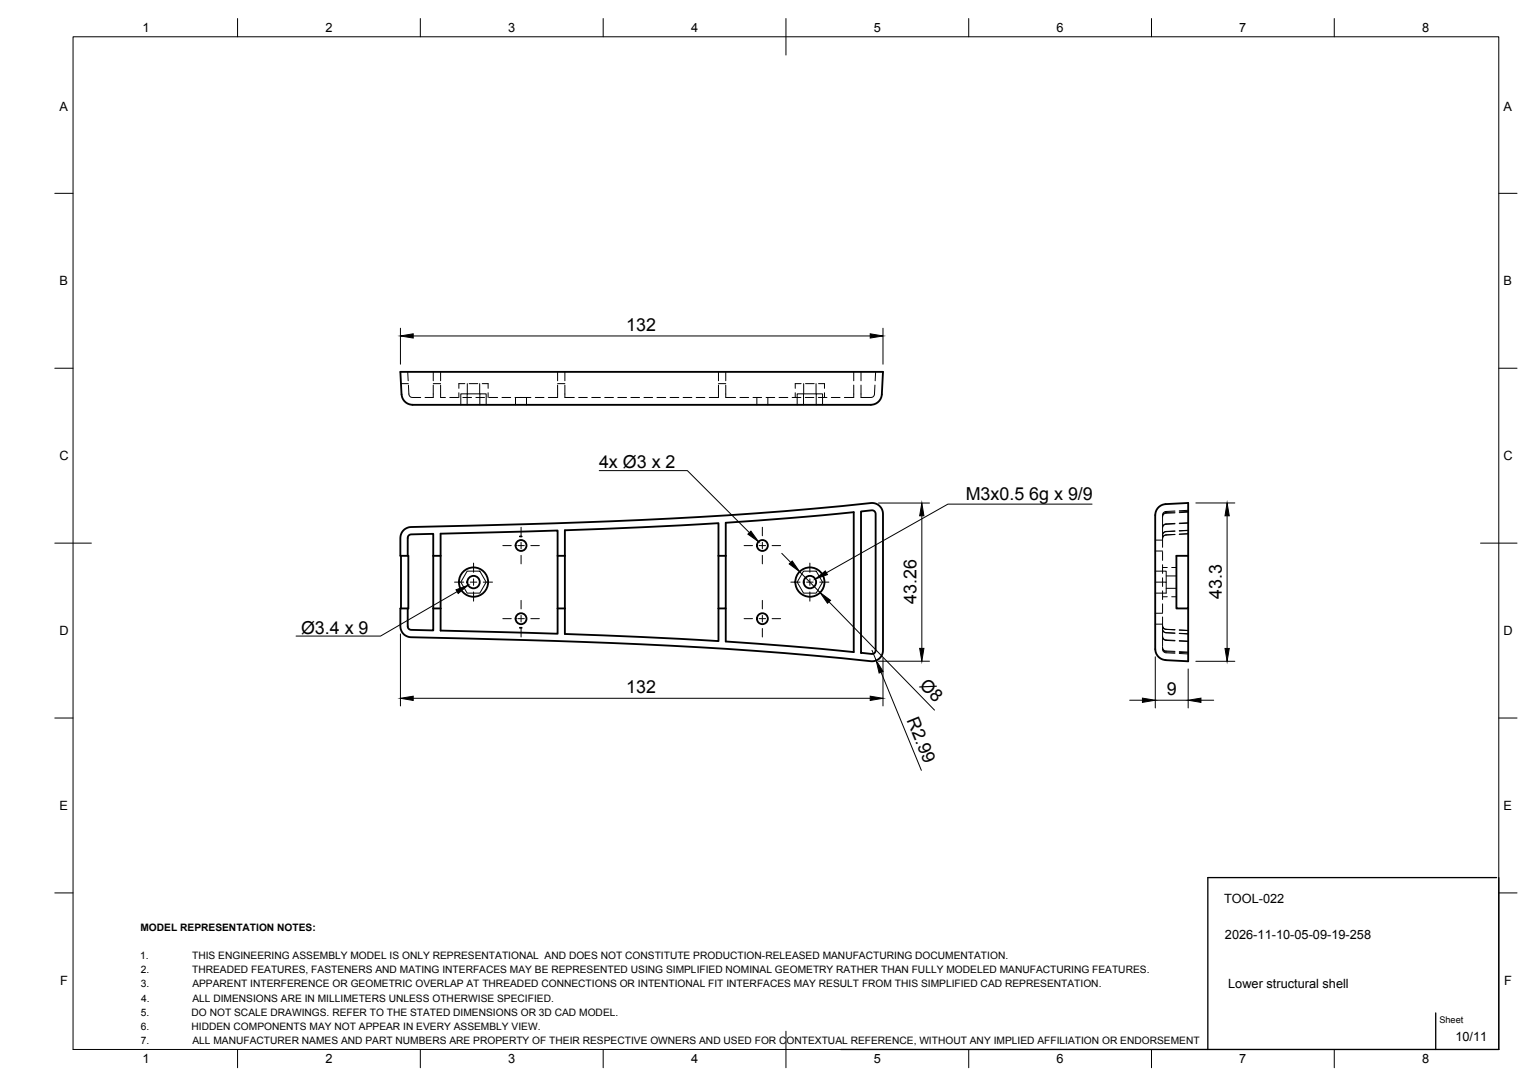
ISO-10303-21;
HEADER;
/* Generated by software containing ST-Developer
 * from STEP Tools, Inc. (www.steptools.com) 
 */

FILE_DESCRIPTION(
/* description */ (''),
/* implementation_level */ '2;1');

FILE_NAME(
/* name */ 'Lower structural shell.step',
/* time_stamp */ '2026-11-10T08:27:36-08:00',
/* author */ (''),
/* organization */ (''),
/* preprocessor_version */ 'ST-DEVELOPER v20.2',
/* originating_system */ 'Autodesk Translation Framework v15.17.0.0',
/* authorisation */ '');

FILE_SCHEMA (('AUTOMOTIVE_DESIGN { 1 0 10303 214 3 1 1 }'));
ENDSEC;

DATA;
#10=MECHANICAL_DESIGN_GEOMETRIC_PRESENTATION_REPRESENTATION('',(#571),#19090);
#84=SPHERICAL_SURFACE('',#7214,0.0999999999999999);
#85=SPHERICAL_SURFACE('',#7217,0.0999999999999997);
#86=SPHERICAL_SURFACE('',#7221,0.0999999999999998);
#87=SPHERICAL_SURFACE('',#7225,0.1);
#88=SPHERICAL_SURFACE('',#7230,0.3);
#89=SPHERICAL_SURFACE('',#7234,0.3);
#90=SPHERICAL_SURFACE('',#7238,0.3);
#91=SPHERICAL_SURFACE('',#7243,0.3);
#124=B_SPLINE_SURFACE_WITH_KNOTS('',3,3,((#12291,#12292,#12293,#12294),
(#12295,#12296,#12297,#12298),(#12299,#12300,#12301,#12302),(#12303,#12304,
#12305,#12306)),.UNSPECIFIED.,.F.,.F.,.F.,(4,4),(4,4),(0.0600191787356395,
0.326709122771036),(0.0105314009467253,0.683686938235975),.UNSPECIFIED.);
#125=B_SPLINE_SURFACE_WITH_KNOTS('',3,3,((#12311,#12312,#12313,#12314),
(#12315,#12316,#12317,#12318),(#12319,#12320,#12321,#12322),(#12323,#12324,
#12325,#12326)),.UNSPECIFIED.,.F.,.F.,.F.,(4,4),(4,4),(0.0251675824878611,
0.0470055662028096),(0.0103663370325175,0.682341693918943),
 .UNSPECIFIED.);
#126=B_SPLINE_SURFACE_WITH_KNOTS('',3,3,((#12336,#12337,#12338,#12339),
(#12340,#12341,#12342,#12343),(#12344,#12345,#12346,#12347),(#12348,#12349,
#12350,#12351),(#12352,#12353,#12354,#12355)),.UNSPECIFIED.,.F.,.F.,.F.,
(4,1,4),(4,4),(0.,0.571428571428571,1.),(0.796205213256333,4.31873271634551),
 .UNSPECIFIED.);
#127=B_SPLINE_SURFACE_WITH_KNOTS('',3,3,((#12360,#12361,#12362,#12363),
(#12364,#12365,#12366,#12367),(#12368,#12369,#12370,#12371),(#12372,#12373,
#12374,#12375),(#12376,#12377,#12378,#12379)),.UNSPECIFIED.,.F.,.F.,.F.,
(4,1,4),(4,4),(0.,0.571428571428571,1.),(0.335767855111383,0.605460332260614),
 .UNSPECIFIED.);
#128=B_SPLINE_SURFACE_WITH_KNOTS('',3,3,((#12398,#12399,#12400,#12401),
(#12402,#12403,#12404,#12405),(#12406,#12407,#12408,#12409),(#12410,#12411,
#12412,#12413),(#12414,#12415,#12416,#12417)),.UNSPECIFIED.,.F.,.F.,.F.,
(4,1,4),(4,4),(0.,0.571428571428571,1.),(8.8675541747208,12.3900816778099),
 .UNSPECIFIED.);
#129=B_SPLINE_SURFACE_WITH_KNOTS('',3,3,((#12422,#12423,#12424,#12425),
(#12426,#12427,#12428,#12429),(#12430,#12431,#12432,#12433),(#12434,#12435,
#12436,#12437)),.UNSPECIFIED.,.F.,.F.,.F.,(4,4),(4,4),(0.673290877228964,
0.939980821264432),(0.010531400969624,0.683686938235975),.UNSPECIFIED.);
#130=B_SPLINE_SURFACE_WITH_KNOTS('',3,3,((#12438,#12439,#12440,#12441),
(#12442,#12443,#12444,#12445),(#12446,#12447,#12448,#12449),(#12450,#12451,
#12452,#12453)),.UNSPECIFIED.,.F.,.F.,.F.,(4,4),(4,4),(0.952994433797115,
0.974832417512139),(0.0103663370325174,0.682341693895801),.UNSPECIFIED.);
#131=B_SPLINE_SURFACE_WITH_KNOTS('',3,3,((#12537,#12538,#12539,#12540),
(#12541,#12542,#12543,#12544),(#12545,#12546,#12547,#12548),(#12549,#12550,
#12551,#12552)),.UNSPECIFIED.,.F.,.F.,.F.,(4,4),(4,4),(0.341076481775573,
0.660379921919131),(0.0113804342297301,0.684288445414502),.UNSPECIFIED.);
#132=B_SPLINE_SURFACE_WITH_KNOTS('',3,3,((#12557,#12558,#12559,#12560),
(#12561,#12562,#12563,#12564),(#12565,#12566,#12567,#12568),(#12569,#12570,
#12571,#12572),(#12573,#12574,#12575,#12576)),.UNSPECIFIED.,.F.,.F.,.F.,
(4,1,4),(4,4),(0.,0.571428571428571,1.),(4.5128966022766,8.72381854299666),
 .UNSPECIFIED.);
#133=B_SPLINE_SURFACE_WITH_KNOTS('',3,3,((#12586,#12587,#12588,#12589),
(#12590,#12591,#12592,#12593),(#12594,#12595,#12596,#12597),(#12598,#12599,
#12600,#12601),(#12602,#12603,#12604,#12605)),.UNSPECIFIED.,.F.,.F.,.F.,
(4,1,4),(4,4),(0.,0.571428571428571,1.),(4.46246834806959,8.67339028878965),
 .UNSPECIFIED.);
#134=B_SPLINE_SURFACE_WITH_KNOTS('',3,3,((#12610,#12611,#12612,#12613),
(#12614,#12615,#12616,#12617),(#12618,#12619,#12620,#12621),(#12622,#12623,
#12624,#12625)),.UNSPECIFIED.,.F.,.F.,.F.,(4,4),(4,4),(0.33962007808087,
0.658923518224427),(0.0113804342297301,0.68428844541339),.UNSPECIFIED.);
#135=B_SPLINE_SURFACE_WITH_KNOTS('',3,3,((#12697,#12698,#12699,#12700),
(#12701,#12702,#12703,#12704),(#12705,#12706,#12707,#12708),(#12709,#12710,
#12711,#12712)),.UNSPECIFIED.,.F.,.F.,.F.,(4,4),(4,4),(0.67474627241906,
0.91907102854965),(0.0117551961069005,0.684448842095107),.UNSPECIFIED.);
#136=B_SPLINE_SURFACE_WITH_KNOTS('',3,3,((#12717,#12718,#12719,#12720),
(#12721,#12722,#12723,#12724),(#12725,#12726,#12727,#12728),(#12729,#12730,
#12731,#12732),(#12733,#12734,#12735,#12736)),.UNSPECIFIED.,.F.,.F.,.F.,
(4,1,4),(4,4),(0.,0.571428571428571,1.),(8.92068531110742,12.1251256661408),
 .UNSPECIFIED.);
#137=B_SPLINE_SURFACE_WITH_KNOTS('',3,3,((#12737,#12738,#12739,#12740),
(#12741,#12742,#12743,#12744),(#12745,#12746,#12747,#12748),(#12749,#12750,
#12751,#12752),(#12753,#12754,#12755,#12756)),.UNSPECIFIED.,.F.,.F.,.F.,
(4,1,4),(4,4),(0.,0.571428571428571,1.),(1.06116122492545,4.26560157995882),
 .UNSPECIFIED.);
#138=B_SPLINE_SURFACE_WITH_KNOTS('',3,3,((#12761,#12762,#12763,#12764),
(#12765,#12766,#12767,#12768),(#12769,#12770,#12771,#12772),(#12773,#12774,
#12775,#12776)),.UNSPECIFIED.,.F.,.F.,.F.,(4,4),(4,4),(0.0809289714503497,
0.325253727580939),(0.011755196108102,0.684448842095106),.UNSPECIFIED.);
#139=B_SPLINE_SURFACE_WITH_KNOTS('',3,3,((#12851,#12852,#12853,#12854),
(#12855,#12856,#12857,#12858),(#12859,#12860,#12861,#12862),(#12863,#12864,
#12865,#12866)),.UNSPECIFIED.,.F.,.F.,.F.,(4,4),(4,4),(0.932204931312898,
0.977820042778932),(0.0118590921259657,0.68448768567755),.UNSPECIFIED.);
#140=B_SPLINE_SURFACE_WITH_KNOTS('',3,3,((#12876,#12877,#12878,#12879),
(#12880,#12881,#12882,#12883),(#12884,#12885,#12886,#12887),(#12888,#12889,
#12890,#12891),(#12892,#12893,#12894,#12895)),.UNSPECIFIED.,.F.,.F.,.F.,
(4,1,4),(4,4),(0.,0.571428571428571,1.),(12.3228618033436,12.893479658151),
 .UNSPECIFIED.);
#141=B_SPLINE_SURFACE_WITH_KNOTS('',3,3,((#12909,#12910,#12911,#12912),
(#12913,#12914,#12915,#12916),(#12917,#12918,#12919,#12920),(#12921,#12922,
#12923,#12924)),.UNSPECIFIED.,.F.,.F.,.F.,(4,4),(4,4),(0.0221799572210682,
0.0677950686870383),(0.0118590921467069,0.68448768567755),.UNSPECIFIED.);
#142=B_SPLINE_SURFACE_WITH_KNOTS('',3,3,((#12934,#12935,#12936,#12937),
(#12938,#12939,#12940,#12941),(#12942,#12943,#12944,#12945),(#12946,#12947,
#12948,#12949),(#12950,#12951,#12952,#12953)),.UNSPECIFIED.,.F.,.F.,.F.,
(4,1,4),(4,4),(0.,0.571428571428571,1.),(0.29280723291527,0.863425087722636),
 .UNSPECIFIED.);
#143=B_SPLINE_SURFACE_WITH_KNOTS('',3,3,((#12967,#12968,#12969,#12970),
(#12971,#12972,#12973,#12974),(#12975,#12976,#12977,#12978),(#12979,#12980,
#12981,#12982),(#12983,#12984,#12985,#12986)),.UNSPECIFIED.,.F.,.F.,.F.,
(4,1,4),(4,4),(0.,0.571428571428571,1.),(0.00866835330220971,0.617725317592517),
 .UNSPECIFIED.);
#144=B_SPLINE_SURFACE_WITH_KNOTS('',3,3,((#12993,#12994,#12995,#12996),
(#12997,#12998,#12999,#13000),(#13001,#13002,#13003,#13004),(#13005,#13006,
#13007,#13008),(#13009,#13010,#13011,#13012),(#13013,#13014,#13015,#13016)),
 .UNSPECIFIED.,.F.,.F.,.F.,(4,1,1,4),(4,4),(0.,0.285714285714286,0.571428571428571,
1.),(0.00654045782928703,0.615688454110788),.UNSPECIFIED.);
#145=B_SPLINE_SURFACE_WITH_KNOTS('',3,3,((#13021,#13022,#13023,#13024),
(#13025,#13026,#13027,#13028),(#13029,#13030,#13031,#13032),(#13033,#13034,
#13035,#13036),(#13037,#13038,#13039,#13040),(#13041,#13042,#13043,#13044)),
 .UNSPECIFIED.,.F.,.F.,.F.,(4,1,1,4),(4,4),(0.,0.285714285714286,0.571428571428571,
1.),(0.00659363931523289,0.615688454110787),.UNSPECIFIED.);
#146=B_SPLINE_SURFACE_WITH_KNOTS('',3,3,((#13049,#13050,#13051,#13052),
(#13053,#13054,#13055,#13056),(#13057,#13058,#13059,#13060),(#13061,#13062,
#13063,#13064),(#13065,#13066,#13067,#13068)),.UNSPECIFIED.,.F.,.F.,.F.,
(4,1,4),(4,4),(0.,0.571428571428571,1.),(12.5808265588057,12.8505190359549),
 .UNSPECIFIED.);
#147=B_SPLINE_SURFACE_WITH_KNOTS('',3,3,((#13069,#13070,#13071,#13072),
(#13073,#13074,#13075,#13076),(#13077,#13078,#13079,#13080),(#13081,#13082,
#13083,#13084),(#13085,#13086,#13087,#13088)),.UNSPECIFIED.,.F.,.F.,.F.,
(4,1,4),(4,4),(0.,0.571428571428571,1.),(0.00865878607617127,0.617725317592517),
 .UNSPECIFIED.);
#148=B_SPLINE_SURFACE_WITH_KNOTS('',3,3,((#13114,#13115,#13116,#13117),
(#13118,#13119,#13120,#13121),(#13122,#13123,#13124,#13125),(#13126,#13127,
#13128,#13129),(#13130,#13131,#13132,#13133)),.UNSPECIFIED.,.F.,.F.,.F.,
(4,1,4),(4,4),(0.,0.571428571428571,1.),(-0.00615755989250974,0.617725317592517),
 .UNSPECIFIED.);
#149=B_SPLINE_SURFACE_WITH_KNOTS('',3,3,((#13152,#13153,#13154,#13155,#13156),
(#13157,#13158,#13159,#13160,#13161),(#13162,#13163,#13164,#13165,#13166),
(#13167,#13168,#13169,#13170,#13171),(#13172,#13173,#13174,#13175,#13176)),
 .UNSPECIFIED.,.F.,.F.,.F.,(4,1,4),(4,1,4),(0.,0.571428571428571,1.),(0.335767855111383,
5.71764434212835,12.893479658151),.UNSPECIFIED.);
#150=B_SPLINE_SURFACE_WITH_KNOTS('',3,3,((#13187,#13188,#13189,#13190),
(#13191,#13192,#13193,#13194),(#13195,#13196,#13197,#13198),(#13199,#13200,
#13201,#13202),(#13203,#13204,#13205,#13206),(#13207,#13208,#13209,#13210)),
 .UNSPECIFIED.,.F.,.F.,.F.,(4,1,1,4),(4,4),(0.,0.285714285714286,0.571428571428571,
1.),(-0.00844595120920508,0.615688454110788),.UNSPECIFIED.);
#151=B_SPLINE_SURFACE_WITH_KNOTS('',3,3,((#13219,#13220,#13221,#13222),
(#13223,#13224,#13225,#13226),(#13227,#13228,#13229,#13230),(#13231,#13232,
#13233,#13234),(#13235,#13236,#13237,#13238),(#13239,#13240,#13241,#13242)),
 .UNSPECIFIED.,.F.,.F.,.F.,(4,1,1,4),(4,4),(0.,0.285714285714286,0.571428571428571,
1.),(-0.00828643285111643,0.615688454110787),.UNSPECIFIED.);
#152=B_SPLINE_SURFACE_WITH_KNOTS('',3,3,((#13251,#13252,#13253,#13254,#13255),
(#13256,#13257,#13258,#13259,#13260),(#13261,#13262,#13263,#13264,#13265),
(#13266,#13267,#13268,#13269,#13270),(#13271,#13272,#13273,#13274,#13275)),
 .UNSPECIFIED.,.F.,.F.,.F.,(4,1,4),(4,1,4),(0.,0.571428571428571,1.),(0.29280723291527,
7.4686425489379,12.8505190359549),.UNSPECIFIED.);
#153=B_SPLINE_SURFACE_WITH_KNOTS('',3,3,((#13286,#13287,#13288,#13289),
(#13290,#13291,#13292,#13293),(#13294,#13295,#13296,#13297),(#13298,#13299,
#13300,#13301),(#13302,#13303,#13304,#13305)),.UNSPECIFIED.,.F.,.F.,.F.,
(4,1,4),(4,4),(0.,0.571428571428571,1.),(-0.0061862132014275,0.617725317592517),
 .UNSPECIFIED.);
#154=B_SPLINE_SURFACE_WITH_KNOTS('',3,3,((#13314,#13315,#13316,#13317),
(#13318,#13319,#13320,#13321),(#13322,#13323,#13324,#13325),(#13326,#13327,
#13328,#13329)),.UNSPECIFIED.,.F.,.F.,.F.,(4,4),(4,4),(0.025165545222094,
0.977821881680028),(0.,0.68448768567755),.UNSPECIFIED.);
#155=B_SPLINE_SURFACE_WITH_KNOTS('',3,3,((#13332,#13333,#13334,#13335),
(#13336,#13337,#13338,#13339),(#13340,#13341,#13342,#13343),(#13344,#13345,
#13346,#13347)),.UNSPECIFIED.,.F.,.F.,.F.,(4,4),(4,4),(0.0221781183199723,
0.974834454777906),(0.,0.68448768567755),.UNSPECIFIED.);
#268=B_SPLINE_CURVE_WITH_KNOTS('',3,(#11245,#11246,#11247,#11248),
 .UNSPECIFIED.,.F.,.F.,(4,4),(3.28016616408593,4.26236080300681),
 .UNSPECIFIED.);
#269=B_SPLINE_CURVE_WITH_KNOTS('',3,(#11252,#11253,#11254,#11255),
 .UNSPECIFIED.,.F.,.F.,(4,4),(8.92392608805945,9.90612072688831),
 .UNSPECIFIED.);
#270=B_SPLINE_CURVE_WITH_KNOTS('',3,(#11257,#11258,#11259,#11260,#11261,
#11262,#11263,#11264,#11265,#11266,#11267,#11268,#11269,#11270,#11271,#11272,
#11273,#11274,#11275),.UNSPECIFIED.,.F.,.F.,(4,3,3,3,3,3,4),(-0.050768112872884,
-0.0388528786649772,-0.0311058171716578,-0.0259830388669653,-0.0210744122964195,
-0.0143837148934404,0.),.UNSPECIFIED.);
#271=B_SPLINE_CURVE_WITH_KNOTS('',3,(#11277,#11278,#11279,#11280),
 .UNSPECIFIED.,.F.,.F.,(4,4),(9.9568018127159,12.1251256661408),
 .UNSPECIFIED.);
#272=B_SPLINE_CURVE_WITH_KNOTS('',3,(#11284,#11285,#11286,#11287),
 .UNSPECIFIED.,.F.,.F.,(4,4),(1.06116122492545,3.22948508825557),
 .UNSPECIFIED.);
#273=B_SPLINE_CURVE_WITH_KNOTS('',3,(#11288,#11289,#11290,#11291,#11292,
#11293,#11294,#11295,#11296,#11297,#11298,#11299,#11300,#11301,#11302,#11303,
#11304,#11305,#11306),.UNSPECIFIED.,.F.,.F.,(4,3,3,3,3,3,4),(-0.0507681129736439,
-0.0388528772897764,-0.0311058147321604,-0.0259830361493327,-0.0210744097201194,
-0.0143837130754026,-9.90506278315E-9),.UNSPECIFIED.);
#274=B_SPLINE_CURVE_WITH_KNOTS('',3,(#11514,#11515,#11516,#11517,#11518,
#11519),.UNSPECIFIED.,.F.,.F.,(4,2,4),(-0.605566356596631,-0.303329629920269,
-0.000148729590407126),.UNSPECIFIED.);
#275=B_SPLINE_CURVE_WITH_KNOTS('',3,(#11521,#11522,#11523,#11524,#11525,
#11526,#11527,#11528,#11529,#11530,#11531,#11532,#11533,#11534,#11535,#11536,
#11537,#11538,#11539,#11540,#11541,#11542,#11543,#11544,#11545,#11546,#11547,
#11548),.UNSPECIFIED.,.F.,.F.,(4,3,3,3,3,3,3,3,3,4),(-0.153210533292091,
-0.129383071834804,-0.117098895005168,-0.0931297672424715,-0.0778761857300216,
-0.065564095006876,-0.0417435583396367,-0.038874550231651,-0.0150983388519663,
0.),.UNSPECIFIED.);
#276=B_SPLINE_CURVE_WITH_KNOTS('',3,(#11552,#11553,#11554,#11555,#11556,
#11557,#11558,#11559,#11560,#11561,#11562,#11563,#11564,#11565,#11566,#11567,
#11568,#11569,#11570,#11571,#11572,#11573,#11574,#11575,#11576,#11577,#11578,
#11579),.UNSPECIFIED.,.F.,.F.,(4,3,3,3,3,3,3,3,3,4),(-0.153244081227051,
-0.129493605146206,-0.117970006482883,-0.0941492904140308,-0.0876825809854227,
-0.078828741443105,-0.0548877675055393,-0.0394694906046094,-0.0155984926894347,
0.),.UNSPECIFIED.);
#277=B_SPLINE_CURVE_WITH_KNOTS('',3,(#11580,#11581,#11582,#11583,#11584,
#11585),.UNSPECIFIED.,.F.,.F.,(4,2,4),(-0.606539490527658,-0.303329031627741,
-0.00112184825655631),.UNSPECIFIED.);
#278=B_SPLINE_CURVE_WITH_KNOTS('',3,(#11590,#11591,#11592,#11593,#11594,
#11595),.UNSPECIFIED.,.F.,.F.,(4,2,4),(-0.606785247764818,-0.303663188081886,
-0.00088649083675002),.UNSPECIFIED.);
#279=B_SPLINE_CURVE_WITH_KNOTS('',3,(#11597,#11598,#11599,#11600,#11601,
#11602,#11603,#11604,#11605,#11606,#11607,#11608,#11609,#11610,#11611,#11612,
#11613,#11614,#11615,#11616,#11617,#11618,#11619,#11620,#11621,#11622,#11623,
#11624),.UNSPECIFIED.,.F.,.F.,(4,3,3,3,3,3,3,3,3,4),(-0.15258577077829,
-0.128839317352572,-0.117158786685373,-0.0932148261566644,-0.0780319390000633,
-0.0653676349965338,-0.0415665498371782,-0.0389909618069961,-0.0152059030050533,
0.),.UNSPECIFIED.);
#280=B_SPLINE_CURVE_WITH_KNOTS('',3,(#11628,#11629,#11630,#11631,#11632,
#11633,#11634,#11635,#11636,#11637,#11638,#11639,#11640,#11641,#11642,#11643,
#11644,#11645,#11646,#11647,#11648,#11649,#11650,#11651,#11652,#11653,#11654,
#11655),.UNSPECIFIED.,.F.,.F.,(4,3,3,3,3,3,3,3,3,4),(-0.152596853546747,
-0.128825864440686,-0.115507515430042,-0.0917263797372463,-0.0872428123353572,
-0.0783995504057471,-0.0544835945915644,-0.0392209901554083,-0.0154275313391792,
0.),.UNSPECIFIED.);
#281=B_SPLINE_CURVE_WITH_KNOTS('',3,(#11657,#11658,#11659,#11660,#11661,
#11662),.UNSPECIFIED.,.F.,.F.,(4,2,4),(-0.606440835737524,-0.303663090452391,
-0.000542069086802599),.UNSPECIFIED.);
#282=B_SPLINE_CURVE_WITH_KNOTS('',3,(#11668,#11669,#11670,#11671,#11672,
#11673),.UNSPECIFIED.,.F.,.F.,(4,2,4),(-0.607379220946441,-0.303761646676304,
-0.00124422999587004),.UNSPECIFIED.);
#283=B_SPLINE_CURVE_WITH_KNOTS('',3,(#11675,#11676,#11677,#11678,#11679,
#11680,#11681,#11682,#11683,#11684,#11685,#11686,#11687,#11688,#11689,#11690,
#11691,#11692,#11693,#11694,#11695,#11696,#11697,#11698,#11699,#11700,#11701,
#11702),.UNSPECIFIED.,.F.,.F.,(4,3,3,3,3,3,3,3,3,4),(-0.152287640102895,
-0.128554450486317,-0.115193035178751,-0.0912770810520543,-0.0781028969167454,
-0.0652733399726575,-0.0414820896655672,-0.0390446621366508,-0.0152552334863041,
0.),.UNSPECIFIED.);
#284=B_SPLINE_CURVE_WITH_KNOTS('',3,(#11706,#11707,#11708,#11709,#11710,
#11711,#11712,#11713,#11714,#11715,#11716,#11717,#11718,#11719,#11720,#11721,
#11722,#11723,#11724,#11725,#11726,#11727,#11728,#11729,#11730,#11731,#11732,
#11733),.UNSPECIFIED.,.F.,.F.,(4,3,3,3,3,3,3,3,3,4),(-0.152291020205185,
-0.128517753946702,-0.115248901231919,-0.0914807886786037,-0.0870359119466785,
-0.0782017654295232,-0.054298407767766,-0.03910658747416,-0.0153486482327859,
0.),.UNSPECIFIED.);
#285=B_SPLINE_CURVE_WITH_KNOTS('',3,(#11735,#11736,#11737,#11738,#11739,
#11740),.UNSPECIFIED.,.F.,.F.,(4,2,4),(-0.606279550122448,-0.303761677523001,
-0.000144559171857295),.UNSPECIFIED.);
#286=B_SPLINE_CURVE_WITH_KNOTS('',3,(#11746,#11747,#11748,#11749,#11750,
#11751),.UNSPECIFIED.,.F.,.F.,(4,2,4),(-0.607536685592867,-0.303784463250135,
-0.00133982193348342),.UNSPECIFIED.);
#287=B_SPLINE_CURVE_WITH_KNOTS('',3,(#11752,#11753,#11754,#11755,#11756,
#11757,#11758,#11759,#11760,#11761,#11762,#11763,#11764,#11765,#11766,#11767,
#11768,#11769,#11770,#11771,#11772,#11773,#11774,#11775,#11776,#11777,#11778,
#11779),.UNSPECIFIED.,.F.,.F.,(4,3,3,3,3,3,3,3,3,4),(-0.152217684890348,
-0.128490376540845,-0.11516578527262,-0.091253137134092,-0.0781160865160423,
-0.0652495101170982,-0.0414606291875136,-0.0390546905501479,-0.015263466236765,
0.),.UNSPECIFIED.);
#288=B_SPLINE_CURVE_WITH_KNOTS('',3,(#11781,#11782,#11783,#11784,#11785,
#11786,#11787,#11788,#11789,#11790,#11791,#11792,#11793,#11794,#11795,#11796,
#11797,#11798,#11799,#11800,#11801,#11802,#11803,#11804,#11805,#11806,#11807,
#11808),.UNSPECIFIED.,.F.,.F.,(4,3,3,3,3,3,3,3,3,4),(-0.152219351639196,
-0.128444680332832,-0.115193337419806,-0.0914284185691762,-0.0869890032859244,
-0.0781648487722283,-0.0542647883944502,-0.0390852411900305,-0.0153331469286526,
0.),.UNSPECIFIED.);
#289=B_SPLINE_CURVE_WITH_KNOTS('',3,(#11810,#11811,#11812,#11813,#11814,
#11815),.UNSPECIFIED.,.F.,.F.,(4,2,4),(-0.606231877025315,-0.303784501204342,
-3.50089943914611E-5),.UNSPECIFIED.);
#290=B_SPLINE_CURVE_WITH_KNOTS('',3,(#11821,#11822,#11823,#11824),
 .UNSPECIFIED.,.F.,.F.,(4,4),(0.0108333608245492,0.617725317592517),
 .UNSPECIFIED.);
#291=B_SPLINE_CURVE_WITH_KNOTS('',3,(#11828,#11829,#11830,#11831),
 .UNSPECIFIED.,.F.,.F.,(4,4),(-0.617725317592517,-0.0108333608245492),
 .UNSPECIFIED.);
#292=B_SPLINE_CURVE_WITH_KNOTS('',3,(#11834,#11835,#11836,#11837),
 .UNSPECIFIED.,.F.,.F.,(4,4),(8.65483889175297,12.1899094612697),
 .UNSPECIFIED.);
#293=B_SPLINE_CURVE_WITH_KNOTS('',3,(#11838,#11839,#11840,#11841),
 .UNSPECIFIED.,.F.,.F.,(4,4),(0.491886782059505,4.00844302274363),
 .UNSPECIFIED.);
#294=B_SPLINE_CURVE_WITH_KNOTS('',3,(#11844,#11845,#11846,#11847,#11848,
#11849,#11850,#11851,#11852,#11853),.UNSPECIFIED.,.F.,.F.,(4,3,3,4),(4.20909064274042,
6.3236533433415,8.26419514194387,8.41669725637478),.UNSPECIFIED.);
#295=B_SPLINE_CURVE_WITH_KNOTS('',3,(#11856,#11857,#11858,#11859),
 .UNSPECIFIED.,.F.,.F.,(4,4),(8.61714174069208,11.8187712274298),
 .UNSPECIFIED.);
#296=B_SPLINE_CURVE_WITH_KNOTS('',3,(#11863,#11864,#11865,#11866),
 .UNSPECIFIED.,.F.,.F.,(4,4),(12.0182076143484,12.6179302061492),
 .UNSPECIFIED.);
#297=B_SPLINE_CURVE_WITH_KNOTS('',3,(#11867,#11868,#11869,#11870,#11871,
#11872,#11873,#11874,#11875,#11876,#11877,#11878,#11879,#11880,#11881,#11882,
#11883,#11884,#11885,#11886,#11887,#11888,#11889,#11890,#11891,#11892,#11893,
#11894),.UNSPECIFIED.,.F.,.F.,(4,3,3,3,3,3,3,3,3,4),(0.,0.023812730958415,
0.0390943730497349,0.0628727645281949,0.0664866407211859,0.0780895647789142,
0.102003044086093,0.117056568347941,0.14081843048439,0.155095961761698),
 .UNSPECIFIED.);
#298=B_SPLINE_CURVE_WITH_KNOTS('',3,(#11898,#11899,#11900,#11901,#11902,
#11903,#11904,#11905,#11906,#11907,#11908,#11909,#11910,#11911,#11912,#11913,
#11914,#11915,#11916,#11917,#11918,#11919,#11920,#11921,#11922,#11923,#11924,
#11925,#11926,#11927,#11928,#11929,#11930,#11931,#11932,#11933,#11934),
 .UNSPECIFIED.,.F.,.F.,(4,3,3,3,3,3,3,3,3,3,3,3,4),(0.,0.0535193130531386,
0.107740084455895,0.117281563739951,0.171478196787188,0.199460035548543,
0.234266327019636,0.287962832542679,0.34249270416273,0.351167719367162,
0.408228095477446,0.46132246935065,0.46528847158773),.UNSPECIFIED.);
#299=B_SPLINE_CURVE_WITH_KNOTS('',3,(#11936,#11937,#11938,#11939),
 .UNSPECIFIED.,.F.,.F.,(4,4),(0.0221781183199723,0.974834454777906),
 .UNSPECIFIED.);
#300=B_SPLINE_CURVE_WITH_KNOTS('',3,(#11941,#11942,#11943,#11944,#11945,
#11946,#11947,#11948,#11949,#11950,#11951,#11952,#11953,#11954,#11955,#11956,
#11957,#11958,#11959,#11960,#11961,#11962,#11963,#11964,#11965,#11966,#11967,
#11968,#11969,#11970,#11971,#11972,#11973,#11974,#11975,#11976,#11977,#11978,
#11979,#11980,#11981,#11982,#11983),.UNSPECIFIED.,.F.,.F.,(4,3,3,3,3,3,
3,3,3,3,3,3,3,3,4),(0.,0.0533317239385299,0.107762434368039,0.117305236535198,
0.171635266834242,0.216430402805854,0.234303130921432,0.288010415584935,
0.341932185058889,0.351200358601802,0.360578786332496,0.414653942238971,
0.427906071157934,0.482008506259547,0.504658879840573),.UNSPECIFIED.);
#301=B_SPLINE_CURVE_WITH_KNOTS('',3,(#11987,#11988,#11989,#11990,#11991,
#11992,#11993,#11994,#11995,#11996,#11997,#11998,#11999,#12000,#12001,#12002,
#12003,#12004,#12005,#12006,#12007,#12008,#12009,#12010,#12011,#12012,#12013,
#12014,#12015,#12016,#12017,#12018,#12019,#12020,#12021,#12022,#12023,#12024,
#12025,#12026,#12027,#12028,#12029),.UNSPECIFIED.,.F.,.F.,(4,3,3,3,3,3,
3,3,3,3,3,3,3,3,4),(0.,0.0533492049661439,0.107791770949794,0.117401360885473,
0.171729175646356,0.216477851539682,0.234467324023732,0.288191829779795,
0.342104640447882,0.351366010290958,0.360619117109406,0.414688080797906,
0.427993719046535,0.482081475021072,0.504664253934307),.UNSPECIFIED.);
#302=B_SPLINE_CURVE_WITH_KNOTS('',3,(#12031,#12032,#12033,#12034),
 .UNSPECIFIED.,.F.,.F.,(4,4),(0.0251655452220943,0.977821881680028),
 .UNSPECIFIED.);
#303=B_SPLINE_CURVE_WITH_KNOTS('',3,(#12036,#12037,#12038,#12039,#12040,
#12041,#12042,#12043,#12044,#12045,#12046,#12047,#12048,#12049,#12050,#12051,
#12052,#12053,#12054,#12055,#12056,#12057,#12058,#12059,#12060,#12061,#12062,
#12063,#12064,#12065,#12066,#12067,#12068,#12069,#12070,#12071,#12072),
 .UNSPECIFIED.,.F.,.F.,(4,3,3,3,3,3,3,3,3,3,3,3,4),(0.,0.053523079491772,
0.107745541051727,0.117301531762597,0.171497090450284,0.19946878868074,
0.234298606923062,0.287998861062908,0.34252758042597,0.351197710209308,
0.408243668718811,0.4613343165756,0.465289627228313),.UNSPECIFIED.);
#304=B_SPLINE_CURVE_WITH_KNOTS('',3,(#12075,#12076,#12077,#12078,#12079,
#12080,#12081,#12082,#12083,#12084,#12085,#12086,#12087,#12088,#12089,#12090,
#12091,#12092,#12093,#12094,#12095,#12096,#12097,#12098,#12099,#12100,#12101,
#12102),.UNSPECIFIED.,.F.,.F.,(4,3,3,3,3,3,3,3,3,4),(0.,0.0238139464176845,
0.039101051769884,0.0628789982206146,0.0664894862143964,0.0781003874493316,
0.102014483019035,0.11706667068295,0.140827139970411,0.155096347075245),
 .UNSPECIFIED.);
#305=B_SPLINE_CURVE_WITH_KNOTS('',3,(#12104,#12105,#12106,#12107),
 .UNSPECIFIED.,.F.,.F.,(4,4),(2.42791692093292E-5,0.602904494019558),
 .UNSPECIFIED.);
#306=B_SPLINE_CURVE_WITH_KNOTS('',3,(#12110,#12111,#12112,#12113),
 .UNSPECIFIED.,.F.,.F.,(4,4),(0.8033909285608,4.02187648095927),
 .UNSPECIFIED.);
#307=B_SPLINE_CURVE_WITH_KNOTS('',3,(#12116,#12117,#12118,#12119,#12120,
#12121,#12122,#12123,#12124,#12125),.UNSPECIFIED.,.F.,.F.,(4,3,3,4),(4.22337623295021,
6.17414866693447,6.32726315261627,8.45313487255185),.UNSPECIFIED.);
#308=B_SPLINE_CURVE_WITH_KNOTS('',3,(#12129,#12130,#12131,#12132),
 .UNSPECIFIED.,.F.,.F.,(4,4),(12.3921295467468,12.6843586902602),
 .UNSPECIFIED.);
#309=B_SPLINE_CURVE_WITH_KNOTS('',3,(#12134,#12135,#12136,#12137,#12138,
#12139,#12140,#12141,#12142,#12143,#12144,#12145,#12146,#12147,#12148,#12149,
#12150,#12151,#12152,#12153,#12154,#12155,#12156,#12157,#12158,#12159,#12160,
#12161,#12162,#12163,#12164,#12165,#12166,#12167),.UNSPECIFIED.,.F.,.F.,
(4,3,3,3,3,3,3,3,3,3,3,4),(0.,0.0238043957114055,0.0391346151758438,0.0629652053320384,
0.0721593756253901,0.0781571886687045,0.101948185591131,0.117123476992186,
0.12020682003633,0.142665945482357,0.166389927689249,0.168222194312373),
 .UNSPECIFIED.);
#310=B_SPLINE_CURVE_WITH_KNOTS('',3,(#12171,#12172,#12173,#12174,#12175,
#12176,#12177,#12178,#12179,#12180,#12181,#12182,#12183,#12184,#12185,#12186,
#12187,#12188,#12189,#12190,#12191,#12192,#12193,#12194,#12195,#12196,#12197,
#12198,#12199,#12200,#12201,#12202,#12203,#12204),.UNSPECIFIED.,.F.,.F.,
(4,3,3,3,3,3,3,3,3,3,3,4),(0.,0.023797882907907,0.039102479174454,0.0629340675289177,
0.0721439954475325,0.0781021576199648,0.101891255326939,0.117067721419617,
0.120193732390416,0.142636523050355,0.16636673084783,0.168220399847748),
 .UNSPECIFIED.);
#311=B_SPLINE_CURVE_WITH_KNOTS('',3,(#12206,#12207,#12208,#12209),
 .UNSPECIFIED.,.F.,.F.,(4,4),(2.71213177756024E-5,0.290725780256064),
 .UNSPECIFIED.);
#312=B_SPLINE_CURVE_WITH_KNOTS('',3,(#12219,#12220,#12221,#12222,#12223,
#12224),.UNSPECIFIED.,.F.,.F.,(4,2,4),(-0.6065913737563,-0.303324265158378,
-0.00121210420063977),.UNSPECIFIED.);
#313=B_SPLINE_CURVE_WITH_KNOTS('',3,(#12226,#12227,#12228,#12229,#12230,
#12231),.UNSPECIFIED.,.F.,.F.,(4,2,4),(-0.605468679705391,-0.303324901248498,
-8.9425867424664E-5),.UNSPECIFIED.);
#314=B_SPLINE_CURVE_WITH_KNOTS('',3,(#12233,#12234,#12235,#12236,#12237,
#12238,#12239,#12240,#12241,#12242,#12243,#12244,#12245,#12246,#12247,#12248,
#12249,#12250,#12251,#12252,#12253,#12254,#12255,#12256,#12257,#12258,#12259,
#12260),.UNSPECIFIED.,.F.,.F.,(4,3,3,3,3,3,3,3,3,4),(-0.153261590805415,
-0.129427422483982,-0.117093626371441,-0.093122524304512,-0.077863059046492,
-0.0655799937729104,-0.0417579003169496,-0.0388648221790391,-0.0150894148558222,
0.),.UNSPECIFIED.);
#315=B_SPLINE_CURVE_WITH_KNOTS('',3,(#12263,#12264,#12265,#12266,#12267,
#12268,#12269,#12270,#12271,#12272,#12273,#12274,#12275,#12276,#12277,#12278,
#12279,#12280,#12281,#12282,#12283,#12284,#12285,#12286,#12287,#12288,#12289,
#12290),.UNSPECIFIED.,.F.,.F.,(4,3,3,3,3,3,3,3,3,4),(-0.153296867786173,
-0.129546774976449,-0.118009772088948,-0.0941871764575653,-0.08771862273971,
-0.0788646444725944,-0.0549216410880561,-0.0394902966566095,-0.0156128557692252,
0.),.UNSPECIFIED.);
#316=B_SPLINE_CURVE_WITH_KNOTS('',3,(#12307,#12308,#12309,#12310),
 .UNSPECIFIED.,.F.,.F.,(4,4),(-4.3123055228435,-0.796205213256333),
 .UNSPECIFIED.);
#317=B_SPLINE_CURVE_WITH_KNOTS('',3,(#12328,#12329,#12330,#12331),
 .UNSPECIFIED.,.F.,.F.,(4,4),(-0.594853877716395,-0.335767855111383),
 .UNSPECIFIED.);
#318=B_SPLINE_CURVE_WITH_KNOTS('',3,(#12332,#12333,#12334,#12335),
 .UNSPECIFIED.,.F.,.F.,(4,4),(-0.615688454110788,-0.00935595183171186),
 .UNSPECIFIED.);
#319=B_SPLINE_CURVE_WITH_KNOTS('',3,(#12356,#12357,#12358,#12359),
 .UNSPECIFIED.,.F.,.F.,(4,4),(0.806548880270408,4.31873271634551),
 .UNSPECIFIED.);
#320=B_SPLINE_CURVE_WITH_KNOTS('',3,(#12381,#12382,#12383,#12384),
 .UNSPECIFIED.,.F.,.F.,(4,4),(0.335767855111383,0.605460332260614),
 .UNSPECIFIED.);
#321=B_SPLINE_CURVE_WITH_KNOTS('',3,(#12387,#12388,#12389,#12390),
 .UNSPECIFIED.,.F.,.F.,(4,4),(8.8675541747208,12.379738010796),
 .UNSPECIFIED.);
#322=B_SPLINE_CURVE_WITH_KNOTS('',3,(#12393,#12394,#12395,#12396),
 .UNSPECIFIED.,.F.,.F.,(4,4),(12.5808265588057,12.8505190359549),
 .UNSPECIFIED.);
#323=B_SPLINE_CURVE_WITH_KNOTS('',3,(#12418,#12419,#12420,#12421),
 .UNSPECIFIED.,.F.,.F.,(4,4),(-12.3900816778099,-8.87398136822274),
 .UNSPECIFIED.);
#324=B_SPLINE_CURVE_WITH_KNOTS('',3,(#12455,#12456,#12457,#12458),
 .UNSPECIFIED.,.F.,.F.,(4,4),(0.00935595183171174,0.615688454110787),
 .UNSPECIFIED.);
#325=B_SPLINE_CURVE_WITH_KNOTS('',3,(#12459,#12460,#12461,#12462),
 .UNSPECIFIED.,.F.,.F.,(4,4),(-12.8505190359549,-12.5914330133498),
 .UNSPECIFIED.);
#326=B_SPLINE_CURVE_WITH_KNOTS('',3,(#12465,#12466,#12467,#12468,#12469,
#12470),.UNSPECIFIED.,.F.,.F.,(4,2,4),(-0.606830654194234,-0.303665168982051,
-0.00091389508118378),.UNSPECIFIED.);
#327=B_SPLINE_CURVE_WITH_KNOTS('',3,(#12472,#12473,#12474,#12475,#12476,
#12477,#12478,#12479,#12480,#12481,#12482,#12483,#12484,#12485,#12486,#12487,
#12488,#12489,#12490,#12491,#12492,#12493,#12494,#12495,#12496,#12497,#12498,
#12499),.UNSPECIFIED.,.F.,.F.,(4,3,3,3,3,3,3,3,3,4),(-0.152562937837783,
-0.12881903955137,-0.117160811640917,-0.0932181166800446,-0.0780374575565173,
-0.0653603882662585,-0.0415602279441365,-0.0389951227734853,-0.0152093108541457,
0.),.UNSPECIFIED.);
#328=B_SPLINE_CURVE_WITH_KNOTS('',3,(#12503,#12504,#12505,#12506,#12507,
#12508,#12509,#12510,#12511,#12512,#12513,#12514,#12515,#12516,#12517,#12518,
#12519,#12520,#12521,#12522,#12523,#12524,#12525,#12526,#12527,#12528,#12529,
#12530),.UNSPECIFIED.,.F.,.F.,(4,3,3,3,3,3,3,3,3,4),(-0.152573286042523,
-0.128801685906155,-0.115487540236632,-0.091707628219999,-0.0872268515824704,
-0.07838422198738,-0.0544695788315335,-0.0392121213631617,-0.0154211067806385,
0.),.UNSPECIFIED.);
#329=B_SPLINE_CURVE_WITH_KNOTS('',3,(#12531,#12532,#12533,#12534,#12535,
#12536),.UNSPECIFIED.,.F.,.F.,(4,2,4),(-0.606417229744719,-0.30366508312326,
-0.000500462001714608),.UNSPECIFIED.);
#330=B_SPLINE_CURVE_WITH_KNOTS('',3,(#12553,#12554,#12555,#12556),
 .UNSPECIFIED.,.F.,.F.,(4,4),(-8.7204856127415,-4.5128966022766),
 .UNSPECIFIED.);
#331=B_SPLINE_CURVE_WITH_KNOTS('',3,(#12577,#12578,#12579,#12580),
 .UNSPECIFIED.,.F.,.F.,(4,4),(4.51913891174751,8.72381854299666),
 .UNSPECIFIED.);
#332=B_SPLINE_CURVE_WITH_KNOTS('',3,(#12582,#12583,#12584,#12585),
 .UNSPECIFIED.,.F.,.F.,(4,4),(4.46246834806959,8.66714797931881),
 .UNSPECIFIED.);
#333=B_SPLINE_CURVE_WITH_KNOTS('',3,(#12606,#12607,#12608,#12609),
 .UNSPECIFIED.,.F.,.F.,(4,4),(-8.67339028878965,-4.46580127832475),
 .UNSPECIFIED.);
#334=B_SPLINE_CURVE_WITH_KNOTS('',3,(#12628,#12629,#12630,#12631,#12632,
#12633),.UNSPECIFIED.,.F.,.F.,(4,2,4),(-0.607391644691745,-0.303762155877002,
-0.00125172564267001),.UNSPECIFIED.);
#335=B_SPLINE_CURVE_WITH_KNOTS('',3,(#12634,#12635,#12636,#12637,#12638,
#12639,#12640,#12641,#12642,#12643,#12644,#12645,#12646,#12647,#12648,#12649,
#12650,#12651,#12652,#12653,#12654,#12655,#12656,#12657,#12658,#12659,#12660,
#12661),.UNSPECIFIED.,.F.,.F.,(4,3,3,3,3,3,3,3,3,4),(-0.152281539067936,
-0.12854821222061,-0.115190816126163,-0.0912758856104041,-0.0781043161616985,
-0.0652713841318381,-0.0414808619979686,-0.039045740680325,-0.0152551599791835,
0.),.UNSPECIFIED.);
#336=B_SPLINE_CURVE_WITH_KNOTS('',3,(#12663,#12664,#12665,#12666,#12667,
#12668,#12669,#12670,#12671,#12672,#12673,#12674,#12675,#12676,#12677,#12678,
#12679,#12680,#12681,#12682,#12683,#12684,#12685,#12686,#12687,#12688,#12689,
#12690),.UNSPECIFIED.,.F.,.F.,(4,3,3,3,3,3,3,3,3,4),(-0.152284734818265,
-0.128510300097745,-0.115243636037359,-0.0914764658269932,-0.0870316758632336,
-0.078197793898112,-0.0542955901223581,-0.0391042908842167,-0.0153462458625635,
0.),.UNSPECIFIED.);
#337=B_SPLINE_CURVE_WITH_KNOTS('',3,(#12691,#12692,#12693,#12694,#12695,
#12696),.UNSPECIFIED.,.F.,.F.,(4,2,4),(-0.606273164239037,-0.303762187833104,
-0.000133245189939568),.UNSPECIFIED.);
#338=B_SPLINE_CURVE_WITH_KNOTS('',3,(#12713,#12714,#12715,#12716),
 .UNSPECIFIED.,.F.,.F.,(4,4),(-12.1227852464729,-8.92068531110742),
 .UNSPECIFIED.);
#339=B_SPLINE_CURVE_WITH_KNOTS('',3,(#12757,#12758,#12759,#12760),
 .UNSPECIFIED.,.F.,.F.,(4,4),(-4.26560157995882,-1.06350164459338),
 .UNSPECIFIED.);
#340=B_SPLINE_CURVE_WITH_KNOTS('',3,(#12779,#12780,#12781,#12782,#12783,
#12784),.UNSPECIFIED.,.F.,.F.,(4,2,4),(-0.607545900263938,-0.303784727094449,
-0.00134539382494125),.UNSPECIFIED.);
#341=B_SPLINE_CURVE_WITH_KNOTS('',3,(#12786,#12787,#12788,#12789,#12790,
#12791,#12792,#12793,#12794,#12795,#12796,#12797,#12798,#12799,#12800,#12801,
#12802,#12803,#12804,#12805,#12806,#12807,#12808,#12809,#12810,#12811,#12812,
#12813),.UNSPECIFIED.,.F.,.F.,(4,3,3,3,3,3,3,3,3,4),(-0.152214473108837,
-0.128485298747135,-0.115164309990209,-0.0912534321321267,-0.0781163092888813,
-0.0652482412471129,-0.0414606388666645,-0.0390548598067502,-0.0152611452145655,
0.),.UNSPECIFIED.);
#342=B_SPLINE_CURVE_WITH_KNOTS('',3,(#12817,#12818,#12819,#12820,#12821,
#12822,#12823,#12824,#12825,#12826,#12827,#12828,#12829,#12830,#12831,#12832,
#12833,#12834,#12835,#12836,#12837,#12838,#12839,#12840,#12841,#12842,#12843,
#12844),.UNSPECIFIED.,.F.,.F.,(4,3,3,3,3,3,3,3,3,4),(-0.152216110966007,
-0.128438825687404,-0.115191384846861,-0.0914281188167518,-0.0869870566155827,
-0.0781642271790374,-0.0542662950786889,-0.0390848818783988,-0.0153309789665,
0.),.UNSPECIFIED.);
#343=B_SPLINE_CURVE_WITH_KNOTS('',3,(#12845,#12846,#12847,#12848,#12849,
#12850),.UNSPECIFIED.,.F.,.F.,(4,2,4),(-0.606227037063105,-0.303784766192107,
-2.65251918123988E-5),.UNSPECIFIED.);
#344=B_SPLINE_CURVE_WITH_KNOTS('',3,(#12868,#12869,#12870,#12871),
 .UNSPECIFIED.,.F.,.F.,(4,4),(0.0107208554739345,0.617725317592517),
 .UNSPECIFIED.);
#345=B_SPLINE_CURVE_WITH_KNOTS('',3,(#12872,#12873,#12874,#12875),
 .UNSPECIFIED.,.F.,.F.,(4,4),(-12.893479658151,-12.3228618033436),
 .UNSPECIFIED.);
#346=B_SPLINE_CURVE_WITH_KNOTS('',3,(#12898,#12899,#12900,#12901),
 .UNSPECIFIED.,.F.,.F.,(4,4),(12.3251818525939,12.893479658151),
 .UNSPECIFIED.);
#347=B_SPLINE_CURVE_WITH_KNOTS('',3,(#12905,#12906,#12907,#12908),
 .UNSPECIFIED.,.F.,.F.,(4,4),(0.292807233425235,0.861105038472338),
 .UNSPECIFIED.);
#348=B_SPLINE_CURVE_WITH_KNOTS('',3,(#12926,#12927,#12928,#12929),
 .UNSPECIFIED.,.F.,.F.,(4,4),(-0.863425087722636,-0.29280723291527),
 .UNSPECIFIED.);
#349=B_SPLINE_CURVE_WITH_KNOTS('',3,(#12930,#12931,#12932,#12933),
 .UNSPECIFIED.,.F.,.F.,(4,4),(-0.617725317592517,-0.0107208554739345),
 .UNSPECIFIED.);
#350=B_SPLINE_CURVE_WITH_KNOTS('',3,(#13017,#13018,#13019,#13020),
 .UNSPECIFIED.,.F.,.F.,(4,4),(0.00878563933291533,0.615688454110788),
 .UNSPECIFIED.);
#351=B_SPLINE_CURVE_WITH_KNOTS('',3,(#13045,#13046,#13047,#13048),
 .UNSPECIFIED.,.F.,.F.,(4,4),(-0.615688454110787,-0.00878563933291527),
 .UNSPECIFIED.);
#352=B_SPLINE_CURVE_WITH_KNOTS('',3,(#13134,#13135,#13136,#13137),
 .UNSPECIFIED.,.F.,.F.,(4,4),(-9.62771529167128E-17,0.617725317592517),
 .UNSPECIFIED.);
#353=B_SPLINE_CURVE_WITH_KNOTS('',3,(#13138,#13139,#13140,#13141),
 .UNSPECIFIED.,.F.,.F.,(4,4),(-0.617725317592517,-0.000337488966422091),
 .UNSPECIFIED.);
#354=B_SPLINE_CURVE_WITH_KNOTS('',3,(#13177,#13178,#13179,#13180,#13181),
 .UNSPECIFIED.,.F.,.F.,(4,1,4),(-12.893479658151,-5.71764434212835,-0.335767855111383),
 .UNSPECIFIED.);
#355=B_SPLINE_CURVE_WITH_KNOTS('',3,(#13182,#13183,#13184,#13185,#13186),
 .UNSPECIFIED.,.F.,.F.,(4,1,4),(0.335767855111383,5.71764434212835,12.893479658151),
 .UNSPECIFIED.);
#356=B_SPLINE_CURVE_WITH_KNOTS('',3,(#13211,#13212,#13213,#13214),
 .UNSPECIFIED.,.F.,.F.,(4,4),(-0.00171041937131743,0.615688454110788),
 .UNSPECIFIED.);
#357=B_SPLINE_CURVE_WITH_KNOTS('',3,(#13215,#13216,#13217,#13218),
 .UNSPECIFIED.,.F.,.F.,(4,4),(-0.615688454110788,-3.98826847727851E-7),
 .UNSPECIFIED.);
#358=B_SPLINE_CURVE_WITH_KNOTS('',3,(#13243,#13244,#13245,#13246),
 .UNSPECIFIED.,.F.,.F.,(4,4),(3.98826847219577E-7,0.615688454110787),
 .UNSPECIFIED.);
#359=B_SPLINE_CURVE_WITH_KNOTS('',3,(#13247,#13248,#13249,#13250),
 .UNSPECIFIED.,.F.,.F.,(4,4),(-0.615688454110787,0.0017104193713176),
 .UNSPECIFIED.);
#360=B_SPLINE_CURVE_WITH_KNOTS('',3,(#13276,#13277,#13278,#13279,#13280),
 .UNSPECIFIED.,.F.,.F.,(4,1,4),(-12.8505190359549,-7.4686425489379,-0.29280723291527),
 .UNSPECIFIED.);
#361=B_SPLINE_CURVE_WITH_KNOTS('',3,(#13281,#13282,#13283,#13284,#13285),
 .UNSPECIFIED.,.F.,.F.,(4,1,4),(0.292807233425236,7.4686425489379,12.8505190359549),
 .UNSPECIFIED.);
#362=B_SPLINE_CURVE_WITH_KNOTS('',3,(#13306,#13307,#13308,#13309),
 .UNSPECIFIED.,.F.,.F.,(4,4),(0.000337488966421928,0.617725317592517),
 .UNSPECIFIED.);
#363=B_SPLINE_CURVE_WITH_KNOTS('',3,(#13310,#13311,#13312,#13313),
 .UNSPECIFIED.,.F.,.F.,(4,4),(-0.617725317592517,8.06646416329215E-17),
 .UNSPECIFIED.);
#551=SHAPE_REPRESENTATION_RELATIONSHIP('SRR','None',#19142,#561);
#561=ADVANCED_BREP_SHAPE_REPRESENTATION('',(#581),#19085);
#571=STYLED_ITEM('',(#19203),#581);
#581=MANIFOLD_SOLID_BREP('Body1',#6825);
#618=FACE_BOUND('',#1385,.T.);
#619=FACE_BOUND('',#1386,.T.);
#620=FACE_BOUND('',#1387,.T.);
#621=FACE_BOUND('',#1399,.T.);
#622=FACE_BOUND('',#1407,.T.);
#623=FACE_BOUND('',#1418,.T.);
#624=FACE_BOUND('',#1420,.T.);
#625=FACE_BOUND('',#1432,.T.);
#626=FACE_BOUND('',#1441,.T.);
#627=FACE_BOUND('',#1442,.T.);
#628=FACE_BOUND('',#1443,.T.);
#629=FACE_BOUND('',#1492,.T.);
#630=FACE_BOUND('',#1493,.T.);
#631=FACE_BOUND('',#1494,.T.);
#632=FACE_BOUND('',#1495,.T.);
#633=FACE_BOUND('',#1496,.T.);
#634=FACE_BOUND('',#1497,.T.);
#734=PLANE('',#7144);
#735=PLANE('',#7158);
#736=PLANE('',#7159);
#737=PLANE('',#7160);
#738=PLANE('',#7161);
#739=PLANE('',#7162);
#740=PLANE('',#7163);
#741=PLANE('',#7164);
#742=PLANE('',#7166);
#743=PLANE('',#7167);
#744=PLANE('',#7168);
#745=PLANE('',#7169);
#746=PLANE('',#7170);
#747=PLANE('',#7171);
#748=PLANE('',#7172);
#749=PLANE('',#7178);
#750=PLANE('',#7179);
#751=PLANE('',#7180);
#752=PLANE('',#7181);
#753=PLANE('',#7182);
#754=PLANE('',#7183);
#755=PLANE('',#7184);
#756=PLANE('',#7185);
#757=PLANE('',#7187);
#758=PLANE('',#7189);
#759=PLANE('',#7190);
#760=PLANE('',#7191);
#761=PLANE('',#7192);
#762=PLANE('',#7193);
#763=PLANE('',#7194);
#764=PLANE('',#7195);
#765=PLANE('',#7196);
#766=PLANE('',#7197);
#767=PLANE('',#7198);
#768=PLANE('',#7199);
#769=PLANE('',#7203);
#770=PLANE('',#7205);
#771=PLANE('',#7206);
#772=PLANE('',#7207);
#773=PLANE('',#7208);
#774=PLANE('',#7209);
#775=PLANE('',#7210);
#776=PLANE('',#7212);
#777=PLANE('',#7229);
#778=PLANE('',#7248);
#779=PLANE('',#7249);
#780=PLANE('',#7250);
#964=FACE_OUTER_BOUND('',#1384,.T.);
#965=FACE_OUTER_BOUND('',#1388,.T.);
#966=FACE_OUTER_BOUND('',#1389,.T.);
#967=FACE_OUTER_BOUND('',#1390,.T.);
#968=FACE_OUTER_BOUND('',#1391,.T.);
#969=FACE_OUTER_BOUND('',#1392,.T.);
#970=FACE_OUTER_BOUND('',#1393,.T.);
#971=FACE_OUTER_BOUND('',#1394,.T.);
#972=FACE_OUTER_BOUND('',#1395,.T.);
#973=FACE_OUTER_BOUND('',#1396,.T.);
#974=FACE_OUTER_BOUND('',#1397,.T.);
#975=FACE_OUTER_BOUND('',#1398,.T.);
#976=FACE_OUTER_BOUND('',#1400,.T.);
#977=FACE_OUTER_BOUND('',#1401,.T.);
#978=FACE_OUTER_BOUND('',#1402,.T.);
#979=FACE_OUTER_BOUND('',#1403,.T.);
#980=FACE_OUTER_BOUND('',#1404,.T.);
#981=FACE_OUTER_BOUND('',#1405,.T.);
#982=FACE_OUTER_BOUND('',#1406,.T.);
#983=FACE_OUTER_BOUND('',#1408,.T.);
#984=FACE_OUTER_BOUND('',#1409,.T.);
#985=FACE_OUTER_BOUND('',#1410,.T.);
#986=FACE_OUTER_BOUND('',#1411,.T.);
#987=FACE_OUTER_BOUND('',#1412,.T.);
#988=FACE_OUTER_BOUND('',#1413,.T.);
#989=FACE_OUTER_BOUND('',#1414,.T.);
#990=FACE_OUTER_BOUND('',#1415,.T.);
#991=FACE_OUTER_BOUND('',#1416,.T.);
#992=FACE_OUTER_BOUND('',#1417,.T.);
#993=FACE_OUTER_BOUND('',#1419,.T.);
#994=FACE_OUTER_BOUND('',#1421,.T.);
#995=FACE_OUTER_BOUND('',#1422,.T.);
#996=FACE_OUTER_BOUND('',#1423,.T.);
#997=FACE_OUTER_BOUND('',#1424,.T.);
#998=FACE_OUTER_BOUND('',#1425,.T.);
#999=FACE_OUTER_BOUND('',#1426,.T.);
#1000=FACE_OUTER_BOUND('',#1427,.T.);
#1001=FACE_OUTER_BOUND('',#1428,.T.);
#1002=FACE_OUTER_BOUND('',#1429,.T.);
#1003=FACE_OUTER_BOUND('',#1430,.T.);
#1004=FACE_OUTER_BOUND('',#1431,.T.);
#1005=FACE_OUTER_BOUND('',#1433,.T.);
#1006=FACE_OUTER_BOUND('',#1434,.T.);
#1007=FACE_OUTER_BOUND('',#1435,.T.);
#1008=FACE_OUTER_BOUND('',#1436,.T.);
#1009=FACE_OUTER_BOUND('',#1437,.T.);
#1010=FACE_OUTER_BOUND('',#1438,.T.);
#1011=FACE_OUTER_BOUND('',#1439,.T.);
#1012=FACE_OUTER_BOUND('',#1440,.T.);
#1013=FACE_OUTER_BOUND('',#1444,.T.);
#1014=FACE_OUTER_BOUND('',#1445,.T.);
#1015=FACE_OUTER_BOUND('',#1446,.T.);
#1016=FACE_OUTER_BOUND('',#1447,.T.);
#1017=FACE_OUTER_BOUND('',#1448,.T.);
#1018=FACE_OUTER_BOUND('',#1449,.T.);
#1019=FACE_OUTER_BOUND('',#1450,.T.);
#1020=FACE_OUTER_BOUND('',#1451,.T.);
#1021=FACE_OUTER_BOUND('',#1452,.T.);
#1022=FACE_OUTER_BOUND('',#1453,.T.);
#1023=FACE_OUTER_BOUND('',#1454,.T.);
#1024=FACE_OUTER_BOUND('',#1455,.T.);
#1025=FACE_OUTER_BOUND('',#1456,.T.);
#1026=FACE_OUTER_BOUND('',#1457,.T.);
#1027=FACE_OUTER_BOUND('',#1458,.T.);
#1028=FACE_OUTER_BOUND('',#1459,.T.);
#1029=FACE_OUTER_BOUND('',#1460,.T.);
#1030=FACE_OUTER_BOUND('',#1461,.T.);
#1031=FACE_OUTER_BOUND('',#1462,.T.);
#1032=FACE_OUTER_BOUND('',#1463,.T.);
#1033=FACE_OUTER_BOUND('',#1464,.T.);
#1034=FACE_OUTER_BOUND('',#1465,.T.);
#1035=FACE_OUTER_BOUND('',#1466,.T.);
#1036=FACE_OUTER_BOUND('',#1467,.T.);
#1037=FACE_OUTER_BOUND('',#1468,.T.);
#1038=FACE_OUTER_BOUND('',#1469,.T.);
#1039=FACE_OUTER_BOUND('',#1470,.T.);
#1040=FACE_OUTER_BOUND('',#1471,.T.);
#1041=FACE_OUTER_BOUND('',#1472,.T.);
#1042=FACE_OUTER_BOUND('',#1473,.T.);
#1043=FACE_OUTER_BOUND('',#1474,.T.);
#1044=FACE_OUTER_BOUND('',#1475,.T.);
#1045=FACE_OUTER_BOUND('',#1476,.T.);
#1046=FACE_OUTER_BOUND('',#1477,.T.);
#1047=FACE_OUTER_BOUND('',#1478,.T.);
#1048=FACE_OUTER_BOUND('',#1479,.T.);
#1049=FACE_OUTER_BOUND('',#1480,.T.);
#1050=FACE_OUTER_BOUND('',#1481,.T.);
#1051=FACE_OUTER_BOUND('',#1482,.T.);
#1052=FACE_OUTER_BOUND('',#1483,.T.);
#1053=FACE_OUTER_BOUND('',#1484,.T.);
#1054=FACE_OUTER_BOUND('',#1485,.T.);
#1055=FACE_OUTER_BOUND('',#1486,.T.);
#1056=FACE_OUTER_BOUND('',#1487,.T.);
#1057=FACE_OUTER_BOUND('',#1488,.T.);
#1058=FACE_OUTER_BOUND('',#1489,.T.);
#1059=FACE_OUTER_BOUND('',#1490,.T.);
#1060=FACE_OUTER_BOUND('',#1491,.T.);
#1061=FACE_OUTER_BOUND('',#1498,.T.);
#1062=FACE_OUTER_BOUND('',#1499,.T.);
#1384=EDGE_LOOP('',(#5085,#5086,#5087,#5088,#5089,#5090,#5091,#5092));
#1385=EDGE_LOOP('',(#5093));
#1386=EDGE_LOOP('',(#5094));
#1387=EDGE_LOOP('',(#5095));
#1388=EDGE_LOOP('',(#5096,#5097,#5098,#5099));
#1389=EDGE_LOOP('',(#5100,#5101,#5102,#5103));
#1390=EDGE_LOOP('',(#5104,#5105,#5106,#5107));
#1391=EDGE_LOOP('',(#5108,#5109,#5110,#5111));
#1392=EDGE_LOOP('',(#5112,#5113,#5114,#5115));
#1393=EDGE_LOOP('',(#5116,#5117,#5118,#5119));
#1394=EDGE_LOOP('',(#5120,#5121,#5122,#5123));
#1395=EDGE_LOOP('',(#5124,#5125,#5126,#5127));
#1396=EDGE_LOOP('',(#5128,#5129,#5130,#5131));
#1397=EDGE_LOOP('',(#5132,#5133,#5134,#5135));
#1398=EDGE_LOOP('',(#5136,#5137,#5138,#5139,#5140,#5141));
#1399=EDGE_LOOP('',(#5142));
#1400=EDGE_LOOP('',(#5143,#5144,#5145,#5146));
#1401=EDGE_LOOP('',(#5147,#5148,#5149,#5150));
#1402=EDGE_LOOP('',(#5151,#5152,#5153,#5154));
#1403=EDGE_LOOP('',(#5155,#5156,#5157,#5158));
#1404=EDGE_LOOP('',(#5159,#5160,#5161,#5162));
#1405=EDGE_LOOP('',(#5163,#5164,#5165,#5166));
#1406=EDGE_LOOP('',(#5167,#5168,#5169,#5170,#5171,#5172));
#1407=EDGE_LOOP('',(#5173));
#1408=EDGE_LOOP('',(#5174,#5175,#5176,#5177));
#1409=EDGE_LOOP('',(#5178,#5179,#5180,#5181));
#1410=EDGE_LOOP('',(#5182,#5183,#5184,#5185));
#1411=EDGE_LOOP('',(#5186,#5187,#5188,#5189));
#1412=EDGE_LOOP('',(#5190,#5191,#5192,#5193));
#1413=EDGE_LOOP('',(#5194,#5195,#5196,#5197));
#1414=EDGE_LOOP('',(#5198,#5199,#5200,#5201));
#1415=EDGE_LOOP('',(#5202,#5203,#5204,#5205));
#1416=EDGE_LOOP('',(#5206,#5207,#5208,#5209));
#1417=EDGE_LOOP('',(#5210));
#1418=EDGE_LOOP('',(#5211));
#1419=EDGE_LOOP('',(#5212));
#1420=EDGE_LOOP('',(#5213));
#1421=EDGE_LOOP('',(#5214,#5215,#5216,#5217));
#1422=EDGE_LOOP('',(#5218,#5219,#5220,#5221));
#1423=EDGE_LOOP('',(#5222,#5223,#5224,#5225));
#1424=EDGE_LOOP('',(#5226,#5227,#5228,#5229));
#1425=EDGE_LOOP('',(#5230,#5231,#5232,#5233));
#1426=EDGE_LOOP('',(#5234,#5235,#5236,#5237,#5238,#5239));
#1427=EDGE_LOOP('',(#5240,#5241,#5242,#5243,#5244,#5245,#5246,#5247,#5248,
#5249));
#1428=EDGE_LOOP('',(#5250,#5251,#5252,#5253,#5254,#5255,#5256,#5257,#5258,
#5259));
#1429=EDGE_LOOP('',(#5260,#5261,#5262,#5263,#5264,#5265,#5266,#5267,#5268,
#5269));
#1430=EDGE_LOOP('',(#5270,#5271,#5272,#5273,#5274,#5275,#5276,#5277));
#1431=EDGE_LOOP('',(#5278,#5279,#5280,#5281,#5282,#5283,#5284,#5285,#5286,
#5287,#5288,#5289,#5290,#5291,#5292,#5293,#5294,#5295,#5296,#5297,#5298,
#5299,#5300,#5301,#5302,#5303,#5304,#5305,#5306,#5307,#5308,#5309,#5310,
#5311,#5312,#5313,#5314,#5315,#5316,#5317,#5318,#5319));
#1432=EDGE_LOOP('',(#5320,#5321,#5322,#5323,#5324,#5325));
#1433=EDGE_LOOP('',(#5326,#5327,#5328,#5329));
#1434=EDGE_LOOP('',(#5330,#5331,#5332,#5333));
#1435=EDGE_LOOP('',(#5334,#5335,#5336,#5337,#5338,#5339));
#1436=EDGE_LOOP('',(#5340,#5341,#5342,#5343));
#1437=EDGE_LOOP('',(#5344,#5345,#5346,#5347));
#1438=EDGE_LOOP('',(#5348,#5349,#5350,#5351));
#1439=EDGE_LOOP('',(#5352,#5353,#5354,#5355));
#1440=EDGE_LOOP('',(#5356,#5357,#5358,#5359));
#1441=EDGE_LOOP('',(#5360));
#1442=EDGE_LOOP('',(#5361));
#1443=EDGE_LOOP('',(#5362));
#1444=EDGE_LOOP('',(#5363,#5364,#5365,#5366));
#1445=EDGE_LOOP('',(#5367,#5368,#5369,#5370));
#1446=EDGE_LOOP('',(#5371,#5372,#5373,#5374));
#1447=EDGE_LOOP('',(#5375,#5376,#5377,#5378));
#1448=EDGE_LOOP('',(#5379,#5380,#5381,#5382,#5383,#5384,#5385,#5386,#5387,
#5388));
#1449=EDGE_LOOP('',(#5389,#5390,#5391,#5392));
#1450=EDGE_LOOP('',(#5393,#5394,#5395,#5396));
#1451=EDGE_LOOP('',(#5397,#5398,#5399,#5400));
#1452=EDGE_LOOP('',(#5401,#5402,#5403,#5404));
#1453=EDGE_LOOP('',(#5405,#5406,#5407,#5408));
#1454=EDGE_LOOP('',(#5409,#5410,#5411,#5412,#5413,#5414,#5415,#5416,#5417,
#5418));
#1455=EDGE_LOOP('',(#5419,#5420,#5421,#5422));
#1456=EDGE_LOOP('',(#5423,#5424,#5425,#5426,#5427,#5428));
#1457=EDGE_LOOP('',(#5429,#5430,#5431,#5432,#5433,#5434));
#1458=EDGE_LOOP('',(#5435,#5436,#5437,#5438));
#1459=EDGE_LOOP('',(#5439,#5440,#5441,#5442,#5443,#5444,#5445,#5446,#5447,
#5448));
#1460=EDGE_LOOP('',(#5449,#5450,#5451,#5452));
#1461=EDGE_LOOP('',(#5453,#5454,#5455,#5456));
#1462=EDGE_LOOP('',(#5457,#5458,#5459,#5460));
#1463=EDGE_LOOP('',(#5461,#5462,#5463,#5464));
#1464=EDGE_LOOP('',(#5465,#5466,#5467,#5468));
#1465=EDGE_LOOP('',(#5469,#5470,#5471));
#1466=EDGE_LOOP('',(#5472,#5473,#5474));
#1467=EDGE_LOOP('',(#5475,#5476,#5477));
#1468=EDGE_LOOP('',(#5478,#5479,#5480,#5481));
#1469=EDGE_LOOP('',(#5482,#5483,#5484,#5485));
#1470=EDGE_LOOP('',(#5486,#5487,#5488));
#1471=EDGE_LOOP('',(#5489,#5490,#5491,#5492));
#1472=EDGE_LOOP('',(#5493,#5494,#5495,#5496));
#1473=EDGE_LOOP('',(#5497,#5498,#5499,#5500));
#1474=EDGE_LOOP('',(#5501,#5502,#5503,#5504));
#1475=EDGE_LOOP('',(#5505,#5506,#5507,#5508));
#1476=EDGE_LOOP('',(#5509,#5510,#5511,#5512));
#1477=EDGE_LOOP('',(#5513,#5514,#5515));
#1478=EDGE_LOOP('',(#5516,#5517,#5518));
#1479=EDGE_LOOP('',(#5519,#5520,#5521));
#1480=EDGE_LOOP('',(#5522,#5523,#5524,#5525));
#1481=EDGE_LOOP('',(#5526,#5527,#5528,#5529));
#1482=EDGE_LOOP('',(#5530,#5531,#5532));
#1483=EDGE_LOOP('',(#5533,#5534,#5535,#5536));
#1484=EDGE_LOOP('',(#5537,#5538,#5539,#5540));
#1485=EDGE_LOOP('',(#5541,#5542,#5543,#5544));
#1486=EDGE_LOOP('',(#5545,#5546,#5547,#5548));
#1487=EDGE_LOOP('',(#5549,#5550,#5551,#5552));
#1488=EDGE_LOOP('',(#5553,#5554,#5555,#5556));
#1489=EDGE_LOOP('',(#5557,#5558,#5559,#5560));
#1490=EDGE_LOOP('',(#5561,#5562,#5563,#5564,#5565,#5566,#5567,#5568));
#1491=EDGE_LOOP('',(#5569,#5570,#5571,#5572));
#1492=EDGE_LOOP('',(#5573,#5574,#5575,#5576,#5577,#5578));
#1493=EDGE_LOOP('',(#5579,#5580,#5581,#5582,#5583,#5584));
#1494=EDGE_LOOP('',(#5585));
#1495=EDGE_LOOP('',(#5586));
#1496=EDGE_LOOP('',(#5587));
#1497=EDGE_LOOP('',(#5588));
#1498=EDGE_LOOP('',(#5589,#5590,#5591,#5592));
#1499=EDGE_LOOP('',(#5593,#5594,#5595,#5596));
#1859=LINE('',#11250,#2308);
#1860=LINE('',#11282,#2309);
#1861=LINE('',#11317,#2310);
#1862=LINE('',#11322,#2311);
#1863=LINE('',#11326,#2312);
#1864=LINE('',#11331,#2313);
#1865=LINE('',#11336,#2314);
#1866=LINE('',#11338,#2315);
#1867=LINE('',#11340,#2316);
#1868=LINE('',#11341,#2317);
#1869=LINE('',#11344,#2318);
#1870=LINE('',#11346,#2319);
#1871=LINE('',#11347,#2320);
#1872=LINE('',#11350,#2321);
#1873=LINE('',#11352,#2322);
#1874=LINE('',#11353,#2323);
#1875=LINE('',#11356,#2324);
#1876=LINE('',#11358,#2325);
#1877=LINE('',#11359,#2326);
#1878=LINE('',#11362,#2327);
#1879=LINE('',#11364,#2328);
#1880=LINE('',#11365,#2329);
#1881=LINE('',#11367,#2330);
#1882=LINE('',#11368,#2331);
#1883=LINE('',#11375,#2332);
#1884=LINE('',#11377,#2333);
#1885=LINE('',#11379,#2334);
#1886=LINE('',#11380,#2335);
#1887=LINE('',#11383,#2336);
#1888=LINE('',#11385,#2337);
#1889=LINE('',#11386,#2338);
#1890=LINE('',#11389,#2339);
#1891=LINE('',#11391,#2340);
#1892=LINE('',#11392,#2341);
#1893=LINE('',#11395,#2342);
#1894=LINE('',#11397,#2343);
#1895=LINE('',#11398,#2344);
#1896=LINE('',#11401,#2345);
#1897=LINE('',#11403,#2346);
#1898=LINE('',#11404,#2347);
#1899=LINE('',#11406,#2348);
#1900=LINE('',#11407,#2349);
#1901=LINE('',#11413,#2350);
#1902=LINE('',#11417,#2351);
#1903=LINE('',#11422,#2352);
#1904=LINE('',#11424,#2353);
#1905=LINE('',#11426,#2354);
#1906=LINE('',#11427,#2355);
#1907=LINE('',#11431,#2356);
#1908=LINE('',#11433,#2357);
#1909=LINE('',#11435,#2358);
#1910=LINE('',#11436,#2359);
#1911=LINE('',#11440,#2360);
#1912=LINE('',#11442,#2361);
#1913=LINE('',#11444,#2362);
#1914=LINE('',#11445,#2363);
#1915=LINE('',#11449,#2364);
#1916=LINE('',#11451,#2365);
#1917=LINE('',#11453,#2366);
#1918=LINE('',#11454,#2367);
#1919=LINE('',#11458,#2368);
#1920=LINE('',#11460,#2369);
#1921=LINE('',#11462,#2370);
#1922=LINE('',#11463,#2371);
#1923=LINE('',#11467,#2372);
#1924=LINE('',#11469,#2373);
#1925=LINE('',#11471,#2374);
#1926=LINE('',#11472,#2375);
#1927=LINE('',#11476,#2376);
#1928=LINE('',#11478,#2377);
#1929=LINE('',#11480,#2378);
#1930=LINE('',#11481,#2379);
#1931=LINE('',#11489,#2380);
#1932=LINE('',#11490,#2381);
#1933=LINE('',#11492,#2382);
#1934=LINE('',#11493,#2383);
#1935=LINE('',#11495,#2384);
#1936=LINE('',#11496,#2385);
#1937=LINE('',#11499,#2386);
#1938=LINE('',#11501,#2387);
#1939=LINE('',#11502,#2388);
#1940=LINE('',#11505,#2389);
#1941=LINE('',#11507,#2390);
#1942=LINE('',#11508,#2391);
#1943=LINE('',#11512,#2392);
#1944=LINE('',#11550,#2393);
#1945=LINE('',#11588,#2394);
#1946=LINE('',#11626,#2395);
#1947=LINE('',#11663,#2396);
#1948=LINE('',#11666,#2397);
#1949=LINE('',#11704,#2398);
#1950=LINE('',#11741,#2399);
#1951=LINE('',#11744,#2400);
#1952=LINE('',#11816,#2401);
#1953=LINE('',#11819,#2402);
#1954=LINE('',#11826,#2403);
#1955=LINE('',#11832,#2404);
#1956=LINE('',#11843,#2405);
#1957=LINE('',#11855,#2406);
#1958=LINE('',#11861,#2407);
#1959=LINE('',#11896,#2408);
#1960=LINE('',#11985,#2409);
#1961=LINE('',#12073,#2410);
#1962=LINE('',#12108,#2411);
#1963=LINE('',#12114,#2412);
#1964=LINE('',#12126,#2413);
#1965=LINE('',#12169,#2414);
#1966=LINE('',#12210,#2415);
#1967=LINE('',#12214,#2416);
#1968=LINE('',#12216,#2417);
#1969=LINE('',#12262,#2418);
#1970=LINE('',#12397,#2419);
#1971=LINE('',#12501,#2420);
#1972=LINE('',#12815,#2421);
#1973=LINE('',#12904,#2422);
#1974=LINE('',#12992,#2423);
#1975=LINE('',#13112,#2424);
#1976=LINE('',#13113,#2425);
#1977=LINE('',#13150,#2426);
#1978=LINE('',#13151,#2427);
#2308=VECTOR('',#8048,1.);
#2309=VECTOR('',#8049,1.);
#2310=VECTOR('',#8060,0.15);
#2311=VECTOR('',#8067,0.15);
#2312=VECTOR('',#8072,0.15);
#2313=VECTOR('',#8077,0.15);
#2314=VECTOR('',#8082,1.);
#2315=VECTOR('',#8083,1.);
#2316=VECTOR('',#8084,1.);
#2317=VECTOR('',#8085,1.);
#2318=VECTOR('',#8088,1.);
#2319=VECTOR('',#8089,1.);
#2320=VECTOR('',#8090,1.);
#2321=VECTOR('',#8093,1.);
#2322=VECTOR('',#8094,1.);
#2323=VECTOR('',#8095,1.);
#2324=VECTOR('',#8098,1.);
#2325=VECTOR('',#8099,1.);
#2326=VECTOR('',#8100,1.);
#2327=VECTOR('',#8103,1.);
#2328=VECTOR('',#8104,1.);
#2329=VECTOR('',#8105,1.);
#2330=VECTOR('',#8108,1.);
#2331=VECTOR('',#8109,1.);
#2332=VECTOR('',#8116,1.);
#2333=VECTOR('',#8117,1.);
#2334=VECTOR('',#8118,1.);
#2335=VECTOR('',#8119,1.);
#2336=VECTOR('',#8122,1.);
#2337=VECTOR('',#8123,1.);
#2338=VECTOR('',#8124,1.);
#2339=VECTOR('',#8127,1.);
#2340=VECTOR('',#8128,1.);
#2341=VECTOR('',#8129,1.);
#2342=VECTOR('',#8132,1.);
#2343=VECTOR('',#8133,1.);
#2344=VECTOR('',#8134,1.);
#2345=VECTOR('',#8137,1.);
#2346=VECTOR('',#8138,1.);
#2347=VECTOR('',#8139,1.);
#2348=VECTOR('',#8142,1.);
#2349=VECTOR('',#8143,1.);
#2350=VECTOR('',#8150,0.17);
#2351=VECTOR('',#8155,0.17);
#2352=VECTOR('',#8160,1.);
#2353=VECTOR('',#8161,1.);
#2354=VECTOR('',#8162,1.);
#2355=VECTOR('',#8163,1.);
#2356=VECTOR('',#8166,1.);
#2357=VECTOR('',#8167,1.);
#2358=VECTOR('',#8168,1.);
#2359=VECTOR('',#8169,1.);
#2360=VECTOR('',#8172,1.);
#2361=VECTOR('',#8173,1.);
#2362=VECTOR('',#8174,1.);
#2363=VECTOR('',#8175,1.);
#2364=VECTOR('',#8178,1.);
#2365=VECTOR('',#8179,1.);
#2366=VECTOR('',#8180,1.);
#2367=VECTOR('',#8181,1.);
#2368=VECTOR('',#8184,1.);
#2369=VECTOR('',#8185,1.);
#2370=VECTOR('',#8186,1.);
#2371=VECTOR('',#8187,1.);
#2372=VECTOR('',#8190,1.);
#2373=VECTOR('',#8191,1.);
#2374=VECTOR('',#8192,1.);
#2375=VECTOR('',#8193,1.);
#2376=VECTOR('',#8196,1.);
#2377=VECTOR('',#8197,1.);
#2378=VECTOR('',#8198,1.);
#2379=VECTOR('',#8199,1.);
#2380=VECTOR('',#8210,1.);
#2381=VECTOR('',#8211,1.);
#2382=VECTOR('',#8214,1.);
#2383=VECTOR('',#8215,1.);
#2384=VECTOR('',#8218,1.);
#2385=VECTOR('',#8219,1.);
#2386=VECTOR('',#8222,1.);
#2387=VECTOR('',#8223,1.);
#2388=VECTOR('',#8224,1.);
#2389=VECTOR('',#8227,1.);
#2390=VECTOR('',#8228,1.);
#2391=VECTOR('',#8229,1.);
#2392=VECTOR('',#8232,1.);
#2393=VECTOR('',#8233,1.);
#2394=VECTOR('',#8236,1.);
#2395=VECTOR('',#8237,1.);
#2396=VECTOR('',#8238,1.);
#2397=VECTOR('',#8241,1.);
#2398=VECTOR('',#8242,1.);
#2399=VECTOR('',#8243,1.);
#2400=VECTOR('',#8246,1.);
#2401=VECTOR('',#8247,1.);
#2402=VECTOR('',#8250,1.);
#2403=VECTOR('',#8251,1.);
#2404=VECTOR('',#8252,1.);
#2405=VECTOR('',#8255,1.);
#2406=VECTOR('',#8256,1.);
#2407=VECTOR('',#8257,1.);
#2408=VECTOR('',#8258,1.);
#2409=VECTOR('',#8259,1.);
#2410=VECTOR('',#8260,1.);
#2411=VECTOR('',#8261,1.);
#2412=VECTOR('',#8262,1.);
#2413=VECTOR('',#8263,1.);
#2414=VECTOR('',#8264,1.);
#2415=VECTOR('',#8265,1.);
#2416=VECTOR('',#8270,0.4);
#2417=VECTOR('',#8273,0.4);
#2418=VECTOR('',#8276,1.);
#2419=VECTOR('',#8283,1.);
#2420=VECTOR('',#8286,1.);
#2421=VECTOR('',#8293,1.);
#2422=VECTOR('',#8298,1.);
#2423=VECTOR('',#8331,1.);
#2424=VECTOR('',#8360,1.);
#2425=VECTOR('',#8361,1.);
#2426=VECTOR('',#8372,1.);
#2427=VECTOR('',#8373,1.);
#2630=CIRCLE('',#7145,0.15);
#2631=CIRCLE('',#7146,0.15);
#2632=CIRCLE('',#7147,0.4);
#2633=CIRCLE('',#7149,0.15);
#2634=CIRCLE('',#7150,0.15);
#2635=CIRCLE('',#7152,0.15);
#2636=CIRCLE('',#7154,0.15);
#2637=CIRCLE('',#7156,0.15);
#2638=CIRCLE('',#7157,0.15);
#2639=CIRCLE('',#7165,0.17);
#2640=CIRCLE('',#7173,0.17);
#2641=CIRCLE('',#7175,0.17);
#2642=CIRCLE('',#7177,0.17);
#2643=CIRCLE('',#7186,0.4);
#2644=CIRCLE('',#7188,0.4);
#2645=CIRCLE('',#7201,0.4);
#2646=CIRCLE('',#7204,0.1);
#2647=CIRCLE('',#7211,0.0999999999999999);
#2648=CIRCLE('',#7213,0.0999999999999999);
#2649=CIRCLE('',#7215,0.0999999999999999);
#2650=CIRCLE('',#7216,0.1);
#2651=CIRCLE('',#7218,0.0999999999999998);
#2652=CIRCLE('',#7219,0.0999999999999998);
#2653=CIRCLE('',#7220,0.0999999999999997);
#2654=CIRCLE('',#7222,0.0999999999999998);
#2655=CIRCLE('',#7223,0.0999999999999998);
#2656=CIRCLE('',#7226,0.0999999999999999);
#2657=CIRCLE('',#7227,0.1);
#2658=CIRCLE('',#7231,0.3);
#2659=CIRCLE('',#7232,0.3);
#2660=CIRCLE('',#7233,0.3);
#2661=CIRCLE('',#7235,0.3);
#2662=CIRCLE('',#7236,0.3);
#2663=CIRCLE('',#7237,0.3);
#2664=CIRCLE('',#7239,0.3);
#2665=CIRCLE('',#7240,0.3);
#2666=CIRCLE('',#7241,0.3);
#2667=CIRCLE('',#7244,0.3);
#2668=CIRCLE('',#7245,0.3);
#2669=CIRCLE('',#7246,0.3);
#2956=VERTEX_POINT('',#11243);
#2957=VERTEX_POINT('',#11244);
#2958=VERTEX_POINT('',#11249);
#2959=VERTEX_POINT('',#11251);
#2960=VERTEX_POINT('',#11256);
#2961=VERTEX_POINT('',#11276);
#2962=VERTEX_POINT('',#11281);
#2963=VERTEX_POINT('',#11283);
#2964=VERTEX_POINT('',#11307);
#2965=VERTEX_POINT('',#11309);
#2966=VERTEX_POINT('',#11311);
#2967=VERTEX_POINT('',#11314);
#2968=VERTEX_POINT('',#11316);
#2969=VERTEX_POINT('',#11320);
#2970=VERTEX_POINT('',#11324);
#2971=VERTEX_POINT('',#11328);
#2972=VERTEX_POINT('',#11330);
#2973=VERTEX_POINT('',#11334);
#2974=VERTEX_POINT('',#11335);
#2975=VERTEX_POINT('',#11337);
#2976=VERTEX_POINT('',#11339);
#2977=VERTEX_POINT('',#11343);
#2978=VERTEX_POINT('',#11345);
#2979=VERTEX_POINT('',#11349);
#2980=VERTEX_POINT('',#11351);
#2981=VERTEX_POINT('',#11355);
#2982=VERTEX_POINT('',#11357);
#2983=VERTEX_POINT('',#11361);
#2984=VERTEX_POINT('',#11363);
#2985=VERTEX_POINT('',#11370);
#2986=VERTEX_POINT('',#11373);
#2987=VERTEX_POINT('',#11374);
#2988=VERTEX_POINT('',#11376);
#2989=VERTEX_POINT('',#11378);
#2990=VERTEX_POINT('',#11382);
#2991=VERTEX_POINT('',#11384);
#2992=VERTEX_POINT('',#11388);
#2993=VERTEX_POINT('',#11390);
#2994=VERTEX_POINT('',#11394);
#2995=VERTEX_POINT('',#11396);
#2996=VERTEX_POINT('',#11400);
#2997=VERTEX_POINT('',#11402);
#2998=VERTEX_POINT('',#11409);
#2999=VERTEX_POINT('',#11412);
#3000=VERTEX_POINT('',#11416);
#3001=VERTEX_POINT('',#11420);
#3002=VERTEX_POINT('',#11421);
#3003=VERTEX_POINT('',#11423);
#3004=VERTEX_POINT('',#11425);
#3005=VERTEX_POINT('',#11429);
#3006=VERTEX_POINT('',#11430);
#3007=VERTEX_POINT('',#11432);
#3008=VERTEX_POINT('',#11434);
#3009=VERTEX_POINT('',#11438);
#3010=VERTEX_POINT('',#11439);
#3011=VERTEX_POINT('',#11441);
#3012=VERTEX_POINT('',#11443);
#3013=VERTEX_POINT('',#11447);
#3014=VERTEX_POINT('',#11448);
#3015=VERTEX_POINT('',#11450);
#3016=VERTEX_POINT('',#11452);
#3017=VERTEX_POINT('',#11456);
#3018=VERTEX_POINT('',#11457);
#3019=VERTEX_POINT('',#11459);
#3020=VERTEX_POINT('',#11461);
#3021=VERTEX_POINT('',#11465);
#3022=VERTEX_POINT('',#11466);
#3023=VERTEX_POINT('',#11468);
#3024=VERTEX_POINT('',#11470);
#3025=VERTEX_POINT('',#11474);
#3026=VERTEX_POINT('',#11475);
#3027=VERTEX_POINT('',#11477);
#3028=VERTEX_POINT('',#11479);
#3029=VERTEX_POINT('',#11483);
#3030=VERTEX_POINT('',#11486);
#3031=VERTEX_POINT('',#11498);
#3032=VERTEX_POINT('',#11500);
#3033=VERTEX_POINT('',#11504);
#3034=VERTEX_POINT('',#11506);
#3035=VERTEX_POINT('',#11510);
#3036=VERTEX_POINT('',#11511);
#3037=VERTEX_POINT('',#11513);
#3038=VERTEX_POINT('',#11520);
#3039=VERTEX_POINT('',#11549);
#3040=VERTEX_POINT('',#11551);
#3041=VERTEX_POINT('',#11587);
#3042=VERTEX_POINT('',#11589);
#3043=VERTEX_POINT('',#11596);
#3044=VERTEX_POINT('',#11625);
#3045=VERTEX_POINT('',#11627);
#3046=VERTEX_POINT('',#11656);
#3047=VERTEX_POINT('',#11665);
#3048=VERTEX_POINT('',#11667);
#3049=VERTEX_POINT('',#11674);
#3050=VERTEX_POINT('',#11703);
#3051=VERTEX_POINT('',#11705);
#3052=VERTEX_POINT('',#11734);
#3053=VERTEX_POINT('',#11743);
#3054=VERTEX_POINT('',#11745);
#3055=VERTEX_POINT('',#11780);
#3056=VERTEX_POINT('',#11809);
#3057=VERTEX_POINT('',#11818);
#3058=VERTEX_POINT('',#11820);
#3059=VERTEX_POINT('',#11825);
#3060=VERTEX_POINT('',#11827);
#3061=VERTEX_POINT('',#11842);
#3062=VERTEX_POINT('',#11854);
#3063=VERTEX_POINT('',#11860);
#3064=VERTEX_POINT('',#11862);
#3065=VERTEX_POINT('',#11895);
#3066=VERTEX_POINT('',#11897);
#3067=VERTEX_POINT('',#11935);
#3068=VERTEX_POINT('',#11940);
#3069=VERTEX_POINT('',#11984);
#3070=VERTEX_POINT('',#11986);
#3071=VERTEX_POINT('',#12030);
#3072=VERTEX_POINT('',#12035);
#3073=VERTEX_POINT('',#12074);
#3074=VERTEX_POINT('',#12103);
#3075=VERTEX_POINT('',#12109);
#3076=VERTEX_POINT('',#12115);
#3077=VERTEX_POINT('',#12127);
#3078=VERTEX_POINT('',#12128);
#3079=VERTEX_POINT('',#12133);
#3080=VERTEX_POINT('',#12168);
#3081=VERTEX_POINT('',#12170);
#3082=VERTEX_POINT('',#12205);
#3083=VERTEX_POINT('',#12212);
#3084=VERTEX_POINT('',#12218);
#3085=VERTEX_POINT('',#12225);
#3086=VERTEX_POINT('',#12232);
#3087=VERTEX_POINT('',#12261);
#3088=VERTEX_POINT('',#12327);
#3089=VERTEX_POINT('',#12380);
#3090=VERTEX_POINT('',#12392);
#3091=VERTEX_POINT('',#12454);
#3092=VERTEX_POINT('',#12464);
#3093=VERTEX_POINT('',#12471);
#3094=VERTEX_POINT('',#12500);
#3095=VERTEX_POINT('',#12502);
#3096=VERTEX_POINT('',#12627);
#3097=VERTEX_POINT('',#12662);
#3098=VERTEX_POINT('',#12778);
#3099=VERTEX_POINT('',#12785);
#3100=VERTEX_POINT('',#12814);
#3101=VERTEX_POINT('',#12816);
#3102=VERTEX_POINT('',#12867);
#3103=VERTEX_POINT('',#12896);
#3104=VERTEX_POINT('',#12903);
#3105=VERTEX_POINT('',#12925);
#3106=VERTEX_POINT('',#12960);
#3107=VERTEX_POINT('',#12988);
#3108=VERTEX_POINT('',#13091);
#3109=VERTEX_POINT('',#13092);
#3110=VERTEX_POINT('',#13094);
#3111=VERTEX_POINT('',#13098);
#3112=VERTEX_POINT('',#13099);
#3113=VERTEX_POINT('',#13101);
#3114=VERTEX_POINT('',#13105);
#3115=VERTEX_POINT('',#13106);
#3116=VERTEX_POINT('',#13108);
#3117=VERTEX_POINT('',#13143);
#3118=VERTEX_POINT('',#13144);
#3119=VERTEX_POINT('',#13146);
#3727=EDGE_CURVE('',#2956,#2957,#268,.T.);
#3728=EDGE_CURVE('',#2957,#2958,#1859,.T.);
#3729=EDGE_CURVE('',#2958,#2959,#269,.T.);
#3730=EDGE_CURVE('',#2960,#2959,#270,.T.);
#3731=EDGE_CURVE('',#2960,#2961,#271,.T.);
#3732=EDGE_CURVE('',#2961,#2962,#1860,.T.);
#3733=EDGE_CURVE('',#2962,#2963,#272,.T.);
#3734=EDGE_CURVE('',#2956,#2963,#273,.T.);
#3735=EDGE_CURVE('',#2964,#2964,#2630,.T.);
#3736=EDGE_CURVE('',#2965,#2965,#2631,.T.);
#3737=EDGE_CURVE('',#2966,#2966,#2632,.T.);
#3738=EDGE_CURVE('',#2967,#2967,#2633,.T.);
#3739=EDGE_CURVE('',#2967,#2968,#1861,.T.);
#3740=EDGE_CURVE('',#2968,#2968,#2634,.T.);
#3741=EDGE_CURVE('',#2969,#2969,#2635,.T.);
#3742=EDGE_CURVE('',#2969,#2965,#1862,.T.);
#3743=EDGE_CURVE('',#2970,#2970,#2636,.T.);
#3744=EDGE_CURVE('',#2970,#2964,#1863,.T.);
#3745=EDGE_CURVE('',#2971,#2971,#2637,.T.);
#3746=EDGE_CURVE('',#2971,#2972,#1864,.T.);
#3747=EDGE_CURVE('',#2972,#2972,#2638,.T.);
#3748=EDGE_CURVE('',#2973,#2974,#1865,.T.);
#3749=EDGE_CURVE('',#2973,#2975,#1866,.T.);
#3750=EDGE_CURVE('',#2975,#2976,#1867,.T.);
#3751=EDGE_CURVE('',#2974,#2976,#1868,.T.);
#3752=EDGE_CURVE('',#2977,#2973,#1869,.T.);
#3753=EDGE_CURVE('',#2977,#2978,#1870,.T.);
#3754=EDGE_CURVE('',#2978,#2975,#1871,.T.);
#3755=EDGE_CURVE('',#2979,#2977,#1872,.T.);
#3756=EDGE_CURVE('',#2979,#2980,#1873,.T.);
#3757=EDGE_CURVE('',#2980,#2978,#1874,.T.);
#3758=EDGE_CURVE('',#2981,#2979,#1875,.T.);
#3759=EDGE_CURVE('',#2981,#2982,#1876,.T.);
#3760=EDGE_CURVE('',#2982,#2980,#1877,.T.);
#3761=EDGE_CURVE('',#2983,#2981,#1878,.T.);
#3762=EDGE_CURVE('',#2983,#2984,#1879,.T.);
#3763=EDGE_CURVE('',#2984,#2982,#1880,.T.);
#3764=EDGE_CURVE('',#2974,#2983,#1881,.T.);
#3765=EDGE_CURVE('',#2976,#2984,#1882,.T.);
#3766=EDGE_CURVE('',#2985,#2985,#2639,.T.);
#3767=EDGE_CURVE('',#2986,#2987,#1883,.T.);
#3768=EDGE_CURVE('',#2986,#2988,#1884,.T.);
#3769=EDGE_CURVE('',#2988,#2989,#1885,.T.);
#3770=EDGE_CURVE('',#2987,#2989,#1886,.T.);
#3771=EDGE_CURVE('',#2990,#2986,#1887,.T.);
#3772=EDGE_CURVE('',#2990,#2991,#1888,.T.);
#3773=EDGE_CURVE('',#2991,#2988,#1889,.T.);
#3774=EDGE_CURVE('',#2992,#2990,#1890,.T.);
#3775=EDGE_CURVE('',#2992,#2993,#1891,.T.);
#3776=EDGE_CURVE('',#2993,#2991,#1892,.T.);
#3777=EDGE_CURVE('',#2994,#2992,#1893,.T.);
#3778=EDGE_CURVE('',#2994,#2995,#1894,.T.);
#3779=EDGE_CURVE('',#2995,#2993,#1895,.T.);
#3780=EDGE_CURVE('',#2996,#2994,#1896,.T.);
#3781=EDGE_CURVE('',#2996,#2997,#1897,.T.);
#3782=EDGE_CURVE('',#2997,#2995,#1898,.T.);
#3783=EDGE_CURVE('',#2987,#2996,#1899,.T.);
#3784=EDGE_CURVE('',#2989,#2997,#1900,.T.);
#3785=EDGE_CURVE('',#2998,#2998,#2640,.T.);
#3786=EDGE_CURVE('',#2998,#2999,#1901,.T.);
#3787=EDGE_CURVE('',#2999,#2999,#2641,.T.);
#3788=EDGE_CURVE('',#2985,#3000,#1902,.T.);
#3789=EDGE_CURVE('',#3000,#3000,#2642,.T.);
#3790=EDGE_CURVE('',#3001,#3002,#1903,.T.);
#3791=EDGE_CURVE('',#3003,#3001,#1904,.T.);
#3792=EDGE_CURVE('',#3004,#3003,#1905,.T.);
#3793=EDGE_CURVE('',#3004,#3002,#1906,.T.);
#3794=EDGE_CURVE('',#3005,#3006,#1907,.T.);
#3795=EDGE_CURVE('',#3005,#3007,#1908,.T.);
#3796=EDGE_CURVE('',#3008,#3007,#1909,.T.);
#3797=EDGE_CURVE('',#3006,#3008,#1910,.T.);
#3798=EDGE_CURVE('',#3009,#3010,#1911,.T.);
#3799=EDGE_CURVE('',#3009,#3011,#1912,.T.);
#3800=EDGE_CURVE('',#3012,#3011,#1913,.T.);
#3801=EDGE_CURVE('',#3010,#3012,#1914,.T.);
#3802=EDGE_CURVE('',#3013,#3014,#1915,.T.);
#3803=EDGE_CURVE('',#3013,#3015,#1916,.T.);
#3804=EDGE_CURVE('',#3016,#3015,#1917,.T.);
#3805=EDGE_CURVE('',#3014,#3016,#1918,.T.);
#3806=EDGE_CURVE('',#3017,#3018,#1919,.T.);
#3807=EDGE_CURVE('',#3017,#3019,#1920,.T.);
#3808=EDGE_CURVE('',#3020,#3019,#1921,.T.);
#3809=EDGE_CURVE('',#3018,#3020,#1922,.T.);
#3810=EDGE_CURVE('',#3021,#3022,#1923,.T.);
#3811=EDGE_CURVE('',#3023,#3021,#1924,.T.);
#3812=EDGE_CURVE('',#3024,#3023,#1925,.T.);
#3813=EDGE_CURVE('',#3024,#3022,#1926,.T.);
#3814=EDGE_CURVE('',#3025,#3026,#1927,.T.);
#3815=EDGE_CURVE('',#3027,#3025,#1928,.T.);
#3816=EDGE_CURVE('',#3028,#3027,#1929,.T.);
#3817=EDGE_CURVE('',#3028,#3026,#1930,.T.);
#3818=EDGE_CURVE('',#3029,#3029,#2643,.T.);
#3819=EDGE_CURVE('',#3030,#3030,#2644,.T.);
#3820=EDGE_CURVE('',#3002,#3017,#1931,.T.);
#3821=EDGE_CURVE('',#3019,#3004,#1932,.T.);
#3822=EDGE_CURVE('',#3022,#3005,#1933,.T.);
#3823=EDGE_CURVE('',#3007,#3024,#1934,.T.);
#3824=EDGE_CURVE('',#3026,#3009,#1935,.T.);
#3825=EDGE_CURVE('',#3011,#3028,#1936,.T.);
#3826=EDGE_CURVE('',#3031,#3013,#1937,.T.);
#3827=EDGE_CURVE('',#3032,#3031,#1938,.T.);
#3828=EDGE_CURVE('',#3015,#3032,#1939,.T.);
#3829=EDGE_CURVE('',#3033,#3031,#1940,.T.);
#3830=EDGE_CURVE('',#3034,#3033,#1941,.T.);
#3831=EDGE_CURVE('',#3032,#3034,#1942,.T.);
#3832=EDGE_CURVE('',#3035,#3036,#1943,.T.);
#3833=EDGE_CURVE('',#3037,#3036,#274,.T.);
#3834=EDGE_CURVE('',#3038,#3037,#275,.T.);
#3835=EDGE_CURVE('',#3039,#3038,#1944,.T.);
#3836=EDGE_CURVE('',#3040,#3039,#276,.T.);
#3837=EDGE_CURVE('',#3035,#3040,#277,.T.);
#3838=EDGE_CURVE('',#3034,#3041,#1945,.T.);
#3839=EDGE_CURVE('',#3042,#3041,#278,.T.);
#3840=EDGE_CURVE('',#3043,#3042,#279,.T.);
#3841=EDGE_CURVE('',#3044,#3043,#1946,.T.);
#3842=EDGE_CURVE('',#3045,#3044,#280,.T.);
#3843=EDGE_CURVE('',#3046,#3045,#281,.T.);
#3844=EDGE_CURVE('',#3046,#3016,#1947,.T.);
#3845=EDGE_CURVE('',#3027,#3047,#1948,.T.);
#3846=EDGE_CURVE('',#3048,#3047,#282,.T.);
#3847=EDGE_CURVE('',#3049,#3048,#283,.T.);
#3848=EDGE_CURVE('',#3050,#3049,#1949,.T.);
#3849=EDGE_CURVE('',#3051,#3050,#284,.T.);
#3850=EDGE_CURVE('',#3052,#3051,#285,.T.);
#3851=EDGE_CURVE('',#3052,#3012,#1950,.T.);
#3852=EDGE_CURVE('',#3023,#3053,#1951,.T.);
#3853=EDGE_CURVE('',#3054,#3053,#286,.T.);
#3854=EDGE_CURVE('',#2962,#3054,#287,.T.);
#3855=EDGE_CURVE('',#3055,#2961,#288,.T.);
#3856=EDGE_CURVE('',#3056,#3055,#289,.T.);
#3857=EDGE_CURVE('',#3056,#3008,#1952,.T.);
#3858=EDGE_CURVE('',#3057,#3018,#1953,.T.);
#3859=EDGE_CURVE('',#3057,#3058,#290,.T.);
#3860=EDGE_CURVE('',#3058,#3059,#1954,.T.);
#3861=EDGE_CURVE('',#3059,#3060,#291,.T.);
#3862=EDGE_CURVE('',#3001,#3060,#1955,.T.);
#3863=EDGE_CURVE('',#3046,#3036,#292,.T.);
#3864=EDGE_CURVE('',#3035,#3041,#293,.T.);
#3865=EDGE_CURVE('',#3061,#3033,#1956,.T.);
#3866=EDGE_CURVE('',#3061,#3047,#294,.T.);
#3867=EDGE_CURVE('',#3062,#3025,#1957,.T.);
#3868=EDGE_CURVE('',#3062,#3053,#295,.T.);
#3869=EDGE_CURVE('',#3063,#3021,#1958,.T.);
#3870=EDGE_CURVE('',#3063,#3064,#296,.T.);
#3871=EDGE_CURVE('',#3064,#3057,#297,.T.);
#3872=EDGE_CURVE('',#3020,#3065,#1959,.T.);
#3873=EDGE_CURVE('',#3066,#3065,#298,.T.);
#3874=EDGE_CURVE('',#3066,#3067,#299,.T.);
#3875=EDGE_CURVE('',#3068,#3067,#300,.T.);
#3876=EDGE_CURVE('',#3068,#3069,#1960,.T.);
#3877=EDGE_CURVE('',#3070,#3069,#301,.T.);
#3878=EDGE_CURVE('',#3070,#3071,#302,.T.);
#3879=EDGE_CURVE('',#3072,#3071,#303,.T.);
#3880=EDGE_CURVE('',#3072,#3003,#1961,.T.);
#3881=EDGE_CURVE('',#3060,#3073,#304,.T.);
#3882=EDGE_CURVE('',#3073,#3074,#305,.T.);
#3883=EDGE_CURVE('',#3006,#3074,#1962,.T.);
#3884=EDGE_CURVE('',#3056,#3075,#306,.T.);
#3885=EDGE_CURVE('',#3010,#3075,#1963,.T.);
#3886=EDGE_CURVE('',#3052,#3076,#307,.T.);
#3887=EDGE_CURVE('',#3014,#3076,#1964,.T.);
#3888=EDGE_CURVE('',#3077,#3078,#308,.T.);
#3889=EDGE_CURVE('',#3078,#3079,#309,.T.);
#3890=EDGE_CURVE('',#3079,#3080,#1965,.T.);
#3891=EDGE_CURVE('',#3080,#3081,#310,.T.);
#3892=EDGE_CURVE('',#3081,#3082,#311,.T.);
#3893=EDGE_CURVE('',#3077,#3082,#1966,.T.);
#3894=EDGE_CURVE('',#3083,#3083,#2645,.T.);
#3895=EDGE_CURVE('',#3083,#3030,#1967,.T.);
#3896=EDGE_CURVE('',#2966,#3029,#1968,.T.);
#3897=EDGE_CURVE('',#3077,#3084,#312,.T.);
#3898=EDGE_CURVE('',#3085,#3082,#313,.T.);
#3899=EDGE_CURVE('',#3086,#3085,#314,.T.);
#3900=EDGE_CURVE('',#3087,#3086,#1969,.T.);
#3901=EDGE_CURVE('',#3084,#3087,#315,.T.);
#3902=EDGE_CURVE('',#3045,#3037,#316,.T.);
#3903=EDGE_CURVE('',#3084,#3088,#317,.T.);
#3904=EDGE_CURVE('',#3088,#3078,#318,.T.);
#3905=EDGE_CURVE('',#3038,#3044,#319,.T.);
#3906=EDGE_CURVE('',#3089,#3087,#320,.T.);
#3907=EDGE_CURVE('',#3088,#3089,#2646,.F.);
#3908=EDGE_CURVE('',#3043,#3039,#321,.T.);
#3909=EDGE_CURVE('',#3086,#3090,#322,.T.);
#3910=EDGE_CURVE('',#3090,#3089,#1970,.T.);
#3911=EDGE_CURVE('',#3040,#3042,#323,.T.);
#3912=EDGE_CURVE('',#3081,#3091,#324,.T.);
#3913=EDGE_CURVE('',#3091,#3085,#325,.T.);
#3914=EDGE_CURVE('',#3092,#3076,#326,.T.);
#3915=EDGE_CURVE('',#3093,#3092,#327,.T.);
#3916=EDGE_CURVE('',#3094,#3093,#1971,.T.);
#3917=EDGE_CURVE('',#3095,#3094,#328,.T.);
#3918=EDGE_CURVE('',#3061,#3095,#329,.T.);
#3919=EDGE_CURVE('',#3051,#3092,#330,.T.);
#3920=EDGE_CURVE('',#3093,#3050,#331,.T.);
#3921=EDGE_CURVE('',#3049,#3094,#332,.T.);
#3922=EDGE_CURVE('',#3095,#3048,#333,.T.);
#3923=EDGE_CURVE('',#3096,#3075,#334,.T.);
#3924=EDGE_CURVE('',#2958,#3096,#335,.T.);
#3925=EDGE_CURVE('',#3097,#2957,#336,.T.);
#3926=EDGE_CURVE('',#3062,#3097,#337,.T.);
#3927=EDGE_CURVE('',#3055,#3096,#338,.T.);
#3928=EDGE_CURVE('',#3097,#3054,#339,.T.);
#3929=EDGE_CURVE('',#3098,#3074,#340,.T.);
#3930=EDGE_CURVE('',#3099,#3098,#341,.T.);
#3931=EDGE_CURVE('',#3100,#3099,#1972,.T.);
#3932=EDGE_CURVE('',#3101,#3100,#342,.T.);
#3933=EDGE_CURVE('',#3063,#3101,#343,.T.);
#3934=EDGE_CURVE('',#3073,#3102,#344,.T.);
#3935=EDGE_CURVE('',#3102,#3098,#345,.T.);
#3936=EDGE_CURVE('',#3103,#3102,#2647,.F.);
#3937=EDGE_CURVE('',#3099,#3103,#346,.T.);
#3938=EDGE_CURVE('',#3103,#3104,#1973,.T.);
#3939=EDGE_CURVE('',#3104,#3100,#347,.T.);
#3940=EDGE_CURVE('',#3101,#3105,#348,.T.);
#3941=EDGE_CURVE('',#3105,#3064,#349,.T.);
#3942=EDGE_CURVE('',#3105,#3104,#2648,.F.);
#3943=EDGE_CURVE('',#3104,#3058,#2649,.F.);
#3944=EDGE_CURVE('',#3058,#3105,#2650,.F.);
#3945=EDGE_CURVE('',#3090,#3091,#2651,.F.);
#3946=EDGE_CURVE('',#3091,#3106,#2652,.F.);
#3947=EDGE_CURVE('',#3106,#3090,#2653,.F.);
#3948=EDGE_CURVE('',#3102,#3059,#2654,.F.);
#3949=EDGE_CURVE('',#3059,#3103,#2655,.F.);
#3950=EDGE_CURVE('',#3107,#3088,#2656,.F.);
#3951=EDGE_CURVE('',#3089,#3107,#2657,.F.);
#3952=EDGE_CURVE('',#3107,#3106,#1974,.T.);
#3953=EDGE_CURVE('',#3079,#3107,#350,.T.);
#3954=EDGE_CURVE('',#3106,#3080,#351,.T.);
#3955=EDGE_CURVE('',#3108,#3109,#2658,.F.);
#3956=EDGE_CURVE('',#3110,#3108,#2659,.F.);
#3957=EDGE_CURVE('',#3109,#3110,#2660,.F.);
#3958=EDGE_CURVE('',#3111,#3112,#2661,.F.);
#3959=EDGE_CURVE('',#3113,#3111,#2662,.F.);
#3960=EDGE_CURVE('',#3112,#3113,#2663,.F.);
#3961=EDGE_CURVE('',#3114,#3115,#2664,.F.);
#3962=EDGE_CURVE('',#3116,#3114,#2665,.F.);
#3963=EDGE_CURVE('',#3115,#3116,#2666,.F.);
#3964=EDGE_CURVE('',#3109,#3116,#1975,.T.);
#3965=EDGE_CURVE('',#3114,#3108,#1976,.T.);
#3966=EDGE_CURVE('',#3071,#3115,#352,.T.);
#3967=EDGE_CURVE('',#3116,#3072,#353,.T.);
#3968=EDGE_CURVE('',#3117,#3118,#2667,.F.);
#3969=EDGE_CURVE('',#3119,#3117,#2668,.F.);
#3970=EDGE_CURVE('',#3118,#3119,#2669,.F.);
#3971=EDGE_CURVE('',#3117,#3113,#1977,.T.);
#3972=EDGE_CURVE('',#3111,#3119,#1978,.T.);
#3973=EDGE_CURVE('',#3115,#3118,#354,.T.);
#3974=EDGE_CURVE('',#3119,#3114,#355,.T.);
#3975=EDGE_CURVE('',#3069,#3117,#356,.T.);
#3976=EDGE_CURVE('',#3118,#3070,#357,.T.);
#3977=EDGE_CURVE('',#3067,#3112,#358,.T.);
#3978=EDGE_CURVE('',#3113,#3068,#359,.T.);
#3979=EDGE_CURVE('',#3112,#3110,#360,.T.);
#3980=EDGE_CURVE('',#3108,#3111,#361,.T.);
#3981=EDGE_CURVE('',#3065,#3109,#362,.T.);
#3982=EDGE_CURVE('',#3110,#3066,#363,.T.);
#5085=ORIENTED_EDGE('',*,*,#3727,.T.);
#5086=ORIENTED_EDGE('',*,*,#3728,.T.);
#5087=ORIENTED_EDGE('',*,*,#3729,.T.);
#5088=ORIENTED_EDGE('',*,*,#3730,.F.);
#5089=ORIENTED_EDGE('',*,*,#3731,.T.);
#5090=ORIENTED_EDGE('',*,*,#3732,.T.);
#5091=ORIENTED_EDGE('',*,*,#3733,.T.);
#5092=ORIENTED_EDGE('',*,*,#3734,.F.);
#5093=ORIENTED_EDGE('',*,*,#3735,.T.);
#5094=ORIENTED_EDGE('',*,*,#3736,.T.);
#5095=ORIENTED_EDGE('',*,*,#3737,.T.);
#5096=ORIENTED_EDGE('',*,*,#3738,.F.);
#5097=ORIENTED_EDGE('',*,*,#3739,.T.);
#5098=ORIENTED_EDGE('',*,*,#3740,.F.);
#5099=ORIENTED_EDGE('',*,*,#3739,.F.);
#5100=ORIENTED_EDGE('',*,*,#3741,.F.);
#5101=ORIENTED_EDGE('',*,*,#3742,.T.);
#5102=ORIENTED_EDGE('',*,*,#3736,.F.);
#5103=ORIENTED_EDGE('',*,*,#3742,.F.);
#5104=ORIENTED_EDGE('',*,*,#3743,.F.);
#5105=ORIENTED_EDGE('',*,*,#3744,.T.);
#5106=ORIENTED_EDGE('',*,*,#3735,.F.);
#5107=ORIENTED_EDGE('',*,*,#3744,.F.);
#5108=ORIENTED_EDGE('',*,*,#3745,.F.);
#5109=ORIENTED_EDGE('',*,*,#3746,.T.);
#5110=ORIENTED_EDGE('',*,*,#3747,.F.);
#5111=ORIENTED_EDGE('',*,*,#3746,.F.);
#5112=ORIENTED_EDGE('',*,*,#3748,.F.);
#5113=ORIENTED_EDGE('',*,*,#3749,.T.);
#5114=ORIENTED_EDGE('',*,*,#3750,.T.);
#5115=ORIENTED_EDGE('',*,*,#3751,.F.);
#5116=ORIENTED_EDGE('',*,*,#3752,.F.);
#5117=ORIENTED_EDGE('',*,*,#3753,.T.);
#5118=ORIENTED_EDGE('',*,*,#3754,.T.);
#5119=ORIENTED_EDGE('',*,*,#3749,.F.);
#5120=ORIENTED_EDGE('',*,*,#3755,.F.);
#5121=ORIENTED_EDGE('',*,*,#3756,.T.);
#5122=ORIENTED_EDGE('',*,*,#3757,.T.);
#5123=ORIENTED_EDGE('',*,*,#3753,.F.);
#5124=ORIENTED_EDGE('',*,*,#3758,.F.);
#5125=ORIENTED_EDGE('',*,*,#3759,.T.);
#5126=ORIENTED_EDGE('',*,*,#3760,.T.);
#5127=ORIENTED_EDGE('',*,*,#3756,.F.);
#5128=ORIENTED_EDGE('',*,*,#3761,.F.);
#5129=ORIENTED_EDGE('',*,*,#3762,.T.);
#5130=ORIENTED_EDGE('',*,*,#3763,.T.);
#5131=ORIENTED_EDGE('',*,*,#3759,.F.);
#5132=ORIENTED_EDGE('',*,*,#3764,.F.);
#5133=ORIENTED_EDGE('',*,*,#3751,.T.);
#5134=ORIENTED_EDGE('',*,*,#3765,.T.);
#5135=ORIENTED_EDGE('',*,*,#3762,.F.);
#5136=ORIENTED_EDGE('',*,*,#3765,.F.);
#5137=ORIENTED_EDGE('',*,*,#3750,.F.);
#5138=ORIENTED_EDGE('',*,*,#3754,.F.);
#5139=ORIENTED_EDGE('',*,*,#3757,.F.);
#5140=ORIENTED_EDGE('',*,*,#3760,.F.);
#5141=ORIENTED_EDGE('',*,*,#3763,.F.);
#5142=ORIENTED_EDGE('',*,*,#3766,.F.);
#5143=ORIENTED_EDGE('',*,*,#3767,.F.);
#5144=ORIENTED_EDGE('',*,*,#3768,.T.);
#5145=ORIENTED_EDGE('',*,*,#3769,.T.);
#5146=ORIENTED_EDGE('',*,*,#3770,.F.);
#5147=ORIENTED_EDGE('',*,*,#3771,.F.);
#5148=ORIENTED_EDGE('',*,*,#3772,.T.);
#5149=ORIENTED_EDGE('',*,*,#3773,.T.);
#5150=ORIENTED_EDGE('',*,*,#3768,.F.);
#5151=ORIENTED_EDGE('',*,*,#3774,.F.);
#5152=ORIENTED_EDGE('',*,*,#3775,.T.);
#5153=ORIENTED_EDGE('',*,*,#3776,.T.);
#5154=ORIENTED_EDGE('',*,*,#3772,.F.);
#5155=ORIENTED_EDGE('',*,*,#3777,.F.);
#5156=ORIENTED_EDGE('',*,*,#3778,.T.);
#5157=ORIENTED_EDGE('',*,*,#3779,.T.);
#5158=ORIENTED_EDGE('',*,*,#3775,.F.);
#5159=ORIENTED_EDGE('',*,*,#3780,.F.);
#5160=ORIENTED_EDGE('',*,*,#3781,.T.);
#5161=ORIENTED_EDGE('',*,*,#3782,.T.);
#5162=ORIENTED_EDGE('',*,*,#3778,.F.);
#5163=ORIENTED_EDGE('',*,*,#3783,.F.);
#5164=ORIENTED_EDGE('',*,*,#3770,.T.);
#5165=ORIENTED_EDGE('',*,*,#3784,.T.);
#5166=ORIENTED_EDGE('',*,*,#3781,.F.);
#5167=ORIENTED_EDGE('',*,*,#3784,.F.);
#5168=ORIENTED_EDGE('',*,*,#3769,.F.);
#5169=ORIENTED_EDGE('',*,*,#3773,.F.);
#5170=ORIENTED_EDGE('',*,*,#3776,.F.);
#5171=ORIENTED_EDGE('',*,*,#3779,.F.);
#5172=ORIENTED_EDGE('',*,*,#3782,.F.);
#5173=ORIENTED_EDGE('',*,*,#3785,.F.);
#5174=ORIENTED_EDGE('',*,*,#3785,.T.);
#5175=ORIENTED_EDGE('',*,*,#3786,.T.);
#5176=ORIENTED_EDGE('',*,*,#3787,.F.);
#5177=ORIENTED_EDGE('',*,*,#3786,.F.);
#5178=ORIENTED_EDGE('',*,*,#3766,.T.);
#5179=ORIENTED_EDGE('',*,*,#3788,.T.);
#5180=ORIENTED_EDGE('',*,*,#3789,.F.);
#5181=ORIENTED_EDGE('',*,*,#3788,.F.);
#5182=ORIENTED_EDGE('',*,*,#3790,.F.);
#5183=ORIENTED_EDGE('',*,*,#3791,.F.);
#5184=ORIENTED_EDGE('',*,*,#3792,.F.);
#5185=ORIENTED_EDGE('',*,*,#3793,.T.);
#5186=ORIENTED_EDGE('',*,*,#3794,.F.);
#5187=ORIENTED_EDGE('',*,*,#3795,.T.);
#5188=ORIENTED_EDGE('',*,*,#3796,.F.);
#5189=ORIENTED_EDGE('',*,*,#3797,.F.);
#5190=ORIENTED_EDGE('',*,*,#3798,.F.);
#5191=ORIENTED_EDGE('',*,*,#3799,.T.);
#5192=ORIENTED_EDGE('',*,*,#3800,.F.);
#5193=ORIENTED_EDGE('',*,*,#3801,.F.);
#5194=ORIENTED_EDGE('',*,*,#3802,.F.);
#5195=ORIENTED_EDGE('',*,*,#3803,.T.);
#5196=ORIENTED_EDGE('',*,*,#3804,.F.);
#5197=ORIENTED_EDGE('',*,*,#3805,.F.);
#5198=ORIENTED_EDGE('',*,*,#3806,.F.);
#5199=ORIENTED_EDGE('',*,*,#3807,.T.);
#5200=ORIENTED_EDGE('',*,*,#3808,.F.);
#5201=ORIENTED_EDGE('',*,*,#3809,.F.);
#5202=ORIENTED_EDGE('',*,*,#3810,.F.);
#5203=ORIENTED_EDGE('',*,*,#3811,.F.);
#5204=ORIENTED_EDGE('',*,*,#3812,.F.);
#5205=ORIENTED_EDGE('',*,*,#3813,.T.);
#5206=ORIENTED_EDGE('',*,*,#3814,.F.);
#5207=ORIENTED_EDGE('',*,*,#3815,.F.);
#5208=ORIENTED_EDGE('',*,*,#3816,.F.);
#5209=ORIENTED_EDGE('',*,*,#3817,.T.);
#5210=ORIENTED_EDGE('',*,*,#3818,.F.);
#5211=ORIENTED_EDGE('',*,*,#3787,.T.);
#5212=ORIENTED_EDGE('',*,*,#3819,.F.);
#5213=ORIENTED_EDGE('',*,*,#3789,.T.);
#5214=ORIENTED_EDGE('',*,*,#3820,.F.);
#5215=ORIENTED_EDGE('',*,*,#3793,.F.);
#5216=ORIENTED_EDGE('',*,*,#3821,.F.);
#5217=ORIENTED_EDGE('',*,*,#3807,.F.);
#5218=ORIENTED_EDGE('',*,*,#3822,.F.);
#5219=ORIENTED_EDGE('',*,*,#3813,.F.);
#5220=ORIENTED_EDGE('',*,*,#3823,.F.);
#5221=ORIENTED_EDGE('',*,*,#3795,.F.);
#5222=ORIENTED_EDGE('',*,*,#3824,.F.);
#5223=ORIENTED_EDGE('',*,*,#3817,.F.);
#5224=ORIENTED_EDGE('',*,*,#3825,.F.);
#5225=ORIENTED_EDGE('',*,*,#3799,.F.);
#5226=ORIENTED_EDGE('',*,*,#3826,.F.);
#5227=ORIENTED_EDGE('',*,*,#3827,.F.);
#5228=ORIENTED_EDGE('',*,*,#3828,.F.);
#5229=ORIENTED_EDGE('',*,*,#3803,.F.);
#5230=ORIENTED_EDGE('',*,*,#3829,.F.);
#5231=ORIENTED_EDGE('',*,*,#3830,.F.);
#5232=ORIENTED_EDGE('',*,*,#3831,.F.);
#5233=ORIENTED_EDGE('',*,*,#3827,.T.);
#5234=ORIENTED_EDGE('',*,*,#3832,.T.);
#5235=ORIENTED_EDGE('',*,*,#3833,.F.);
#5236=ORIENTED_EDGE('',*,*,#3834,.F.);
#5237=ORIENTED_EDGE('',*,*,#3835,.F.);
#5238=ORIENTED_EDGE('',*,*,#3836,.F.);
#5239=ORIENTED_EDGE('',*,*,#3837,.F.);
#5240=ORIENTED_EDGE('',*,*,#3804,.T.);
#5241=ORIENTED_EDGE('',*,*,#3828,.T.);
#5242=ORIENTED_EDGE('',*,*,#3831,.T.);
#5243=ORIENTED_EDGE('',*,*,#3838,.T.);
#5244=ORIENTED_EDGE('',*,*,#3839,.F.);
#5245=ORIENTED_EDGE('',*,*,#3840,.F.);
#5246=ORIENTED_EDGE('',*,*,#3841,.F.);
#5247=ORIENTED_EDGE('',*,*,#3842,.F.);
#5248=ORIENTED_EDGE('',*,*,#3843,.F.);
#5249=ORIENTED_EDGE('',*,*,#3844,.T.);
#5250=ORIENTED_EDGE('',*,*,#3800,.T.);
#5251=ORIENTED_EDGE('',*,*,#3825,.T.);
#5252=ORIENTED_EDGE('',*,*,#3816,.T.);
#5253=ORIENTED_EDGE('',*,*,#3845,.T.);
#5254=ORIENTED_EDGE('',*,*,#3846,.F.);
#5255=ORIENTED_EDGE('',*,*,#3847,.F.);
#5256=ORIENTED_EDGE('',*,*,#3848,.F.);
#5257=ORIENTED_EDGE('',*,*,#3849,.F.);
#5258=ORIENTED_EDGE('',*,*,#3850,.F.);
#5259=ORIENTED_EDGE('',*,*,#3851,.T.);
#5260=ORIENTED_EDGE('',*,*,#3796,.T.);
#5261=ORIENTED_EDGE('',*,*,#3823,.T.);
#5262=ORIENTED_EDGE('',*,*,#3812,.T.);
#5263=ORIENTED_EDGE('',*,*,#3852,.T.);
#5264=ORIENTED_EDGE('',*,*,#3853,.F.);
#5265=ORIENTED_EDGE('',*,*,#3854,.F.);
#5266=ORIENTED_EDGE('',*,*,#3732,.F.);
#5267=ORIENTED_EDGE('',*,*,#3855,.F.);
#5268=ORIENTED_EDGE('',*,*,#3856,.F.);
#5269=ORIENTED_EDGE('',*,*,#3857,.T.);
#5270=ORIENTED_EDGE('',*,*,#3790,.T.);
#5271=ORIENTED_EDGE('',*,*,#3820,.T.);
#5272=ORIENTED_EDGE('',*,*,#3806,.T.);
#5273=ORIENTED_EDGE('',*,*,#3858,.F.);
#5274=ORIENTED_EDGE('',*,*,#3859,.T.);
#5275=ORIENTED_EDGE('',*,*,#3860,.T.);
#5276=ORIENTED_EDGE('',*,*,#3861,.T.);
#5277=ORIENTED_EDGE('',*,*,#3862,.F.);
#5278=ORIENTED_EDGE('',*,*,#3805,.T.);
#5279=ORIENTED_EDGE('',*,*,#3844,.F.);
#5280=ORIENTED_EDGE('',*,*,#3863,.T.);
#5281=ORIENTED_EDGE('',*,*,#3832,.F.);
#5282=ORIENTED_EDGE('',*,*,#3864,.T.);
#5283=ORIENTED_EDGE('',*,*,#3838,.F.);
#5284=ORIENTED_EDGE('',*,*,#3830,.T.);
#5285=ORIENTED_EDGE('',*,*,#3865,.F.);
#5286=ORIENTED_EDGE('',*,*,#3866,.T.);
#5287=ORIENTED_EDGE('',*,*,#3845,.F.);
#5288=ORIENTED_EDGE('',*,*,#3815,.T.);
#5289=ORIENTED_EDGE('',*,*,#3867,.F.);
#5290=ORIENTED_EDGE('',*,*,#3868,.T.);
#5291=ORIENTED_EDGE('',*,*,#3852,.F.);
#5292=ORIENTED_EDGE('',*,*,#3811,.T.);
#5293=ORIENTED_EDGE('',*,*,#3869,.F.);
#5294=ORIENTED_EDGE('',*,*,#3870,.T.);
#5295=ORIENTED_EDGE('',*,*,#3871,.T.);
#5296=ORIENTED_EDGE('',*,*,#3858,.T.);
#5297=ORIENTED_EDGE('',*,*,#3809,.T.);
#5298=ORIENTED_EDGE('',*,*,#3872,.T.);
#5299=ORIENTED_EDGE('',*,*,#3873,.F.);
#5300=ORIENTED_EDGE('',*,*,#3874,.T.);
#5301=ORIENTED_EDGE('',*,*,#3875,.F.);
#5302=ORIENTED_EDGE('',*,*,#3876,.T.);
#5303=ORIENTED_EDGE('',*,*,#3877,.F.);
#5304=ORIENTED_EDGE('',*,*,#3878,.T.);
#5305=ORIENTED_EDGE('',*,*,#3879,.F.);
#5306=ORIENTED_EDGE('',*,*,#3880,.T.);
#5307=ORIENTED_EDGE('',*,*,#3791,.T.);
#5308=ORIENTED_EDGE('',*,*,#3862,.T.);
#5309=ORIENTED_EDGE('',*,*,#3881,.T.);
#5310=ORIENTED_EDGE('',*,*,#3882,.T.);
#5311=ORIENTED_EDGE('',*,*,#3883,.F.);
#5312=ORIENTED_EDGE('',*,*,#3797,.T.);
#5313=ORIENTED_EDGE('',*,*,#3857,.F.);
#5314=ORIENTED_EDGE('',*,*,#3884,.T.);
#5315=ORIENTED_EDGE('',*,*,#3885,.F.);
#5316=ORIENTED_EDGE('',*,*,#3801,.T.);
#5317=ORIENTED_EDGE('',*,*,#3851,.F.);
#5318=ORIENTED_EDGE('',*,*,#3886,.T.);
#5319=ORIENTED_EDGE('',*,*,#3887,.F.);
#5320=ORIENTED_EDGE('',*,*,#3888,.T.);
#5321=ORIENTED_EDGE('',*,*,#3889,.T.);
#5322=ORIENTED_EDGE('',*,*,#3890,.T.);
#5323=ORIENTED_EDGE('',*,*,#3891,.T.);
#5324=ORIENTED_EDGE('',*,*,#3892,.T.);
#5325=ORIENTED_EDGE('',*,*,#3893,.F.);
#5326=ORIENTED_EDGE('',*,*,#3894,.F.);
#5327=ORIENTED_EDGE('',*,*,#3895,.T.);
#5328=ORIENTED_EDGE('',*,*,#3819,.T.);
#5329=ORIENTED_EDGE('',*,*,#3895,.F.);
#5330=ORIENTED_EDGE('',*,*,#3737,.F.);
#5331=ORIENTED_EDGE('',*,*,#3896,.T.);
#5332=ORIENTED_EDGE('',*,*,#3818,.T.);
#5333=ORIENTED_EDGE('',*,*,#3896,.F.);
#5334=ORIENTED_EDGE('',*,*,#3897,.F.);
#5335=ORIENTED_EDGE('',*,*,#3893,.T.);
#5336=ORIENTED_EDGE('',*,*,#3898,.F.);
#5337=ORIENTED_EDGE('',*,*,#3899,.F.);
#5338=ORIENTED_EDGE('',*,*,#3900,.F.);
#5339=ORIENTED_EDGE('',*,*,#3901,.F.);
#5340=ORIENTED_EDGE('',*,*,#3833,.T.);
#5341=ORIENTED_EDGE('',*,*,#3863,.F.);
#5342=ORIENTED_EDGE('',*,*,#3843,.T.);
#5343=ORIENTED_EDGE('',*,*,#3902,.T.);
#5344=ORIENTED_EDGE('',*,*,#3897,.T.);
#5345=ORIENTED_EDGE('',*,*,#3903,.T.);
#5346=ORIENTED_EDGE('',*,*,#3904,.T.);
#5347=ORIENTED_EDGE('',*,*,#3888,.F.);
#5348=ORIENTED_EDGE('',*,*,#3834,.T.);
#5349=ORIENTED_EDGE('',*,*,#3902,.F.);
#5350=ORIENTED_EDGE('',*,*,#3842,.T.);
#5351=ORIENTED_EDGE('',*,*,#3905,.F.);
#5352=ORIENTED_EDGE('',*,*,#3901,.T.);
#5353=ORIENTED_EDGE('',*,*,#3906,.F.);
#5354=ORIENTED_EDGE('',*,*,#3907,.F.);
#5355=ORIENTED_EDGE('',*,*,#3903,.F.);
#5356=ORIENTED_EDGE('',*,*,#3835,.T.);
#5357=ORIENTED_EDGE('',*,*,#3905,.T.);
#5358=ORIENTED_EDGE('',*,*,#3841,.T.);
#5359=ORIENTED_EDGE('',*,*,#3908,.T.);
#5360=ORIENTED_EDGE('',*,*,#3740,.T.);
#5361=ORIENTED_EDGE('',*,*,#3747,.T.);
#5362=ORIENTED_EDGE('',*,*,#3894,.T.);
#5363=ORIENTED_EDGE('',*,*,#3900,.T.);
#5364=ORIENTED_EDGE('',*,*,#3909,.T.);
#5365=ORIENTED_EDGE('',*,*,#3910,.T.);
#5366=ORIENTED_EDGE('',*,*,#3906,.T.);
#5367=ORIENTED_EDGE('',*,*,#3836,.T.);
#5368=ORIENTED_EDGE('',*,*,#3908,.F.);
#5369=ORIENTED_EDGE('',*,*,#3840,.T.);
#5370=ORIENTED_EDGE('',*,*,#3911,.F.);
#5371=ORIENTED_EDGE('',*,*,#3837,.T.);
#5372=ORIENTED_EDGE('',*,*,#3911,.T.);
#5373=ORIENTED_EDGE('',*,*,#3839,.T.);
#5374=ORIENTED_EDGE('',*,*,#3864,.F.);
#5375=ORIENTED_EDGE('',*,*,#3898,.T.);
#5376=ORIENTED_EDGE('',*,*,#3892,.F.);
#5377=ORIENTED_EDGE('',*,*,#3912,.T.);
#5378=ORIENTED_EDGE('',*,*,#3913,.T.);
#5379=ORIENTED_EDGE('',*,*,#3802,.T.);
#5380=ORIENTED_EDGE('',*,*,#3887,.T.);
#5381=ORIENTED_EDGE('',*,*,#3914,.F.);
#5382=ORIENTED_EDGE('',*,*,#3915,.F.);
#5383=ORIENTED_EDGE('',*,*,#3916,.F.);
#5384=ORIENTED_EDGE('',*,*,#3917,.F.);
#5385=ORIENTED_EDGE('',*,*,#3918,.F.);
#5386=ORIENTED_EDGE('',*,*,#3865,.T.);
#5387=ORIENTED_EDGE('',*,*,#3829,.T.);
#5388=ORIENTED_EDGE('',*,*,#3826,.T.);
#5389=ORIENTED_EDGE('',*,*,#3914,.T.);
#5390=ORIENTED_EDGE('',*,*,#3886,.F.);
#5391=ORIENTED_EDGE('',*,*,#3850,.T.);
#5392=ORIENTED_EDGE('',*,*,#3919,.T.);
#5393=ORIENTED_EDGE('',*,*,#3915,.T.);
#5394=ORIENTED_EDGE('',*,*,#3919,.F.);
#5395=ORIENTED_EDGE('',*,*,#3849,.T.);
#5396=ORIENTED_EDGE('',*,*,#3920,.F.);
#5397=ORIENTED_EDGE('',*,*,#3916,.T.);
#5398=ORIENTED_EDGE('',*,*,#3920,.T.);
#5399=ORIENTED_EDGE('',*,*,#3848,.T.);
#5400=ORIENTED_EDGE('',*,*,#3921,.T.);
#5401=ORIENTED_EDGE('',*,*,#3917,.T.);
#5402=ORIENTED_EDGE('',*,*,#3921,.F.);
#5403=ORIENTED_EDGE('',*,*,#3847,.T.);
#5404=ORIENTED_EDGE('',*,*,#3922,.F.);
#5405=ORIENTED_EDGE('',*,*,#3918,.T.);
#5406=ORIENTED_EDGE('',*,*,#3922,.T.);
#5407=ORIENTED_EDGE('',*,*,#3846,.T.);
#5408=ORIENTED_EDGE('',*,*,#3866,.F.);
#5409=ORIENTED_EDGE('',*,*,#3798,.T.);
#5410=ORIENTED_EDGE('',*,*,#3885,.T.);
#5411=ORIENTED_EDGE('',*,*,#3923,.F.);
#5412=ORIENTED_EDGE('',*,*,#3924,.F.);
#5413=ORIENTED_EDGE('',*,*,#3728,.F.);
#5414=ORIENTED_EDGE('',*,*,#3925,.F.);
#5415=ORIENTED_EDGE('',*,*,#3926,.F.);
#5416=ORIENTED_EDGE('',*,*,#3867,.T.);
#5417=ORIENTED_EDGE('',*,*,#3814,.T.);
#5418=ORIENTED_EDGE('',*,*,#3824,.T.);
#5419=ORIENTED_EDGE('',*,*,#3923,.T.);
#5420=ORIENTED_EDGE('',*,*,#3884,.F.);
#5421=ORIENTED_EDGE('',*,*,#3856,.T.);
#5422=ORIENTED_EDGE('',*,*,#3927,.T.);
#5423=ORIENTED_EDGE('',*,*,#3730,.T.);
#5424=ORIENTED_EDGE('',*,*,#3729,.F.);
#5425=ORIENTED_EDGE('',*,*,#3924,.T.);
#5426=ORIENTED_EDGE('',*,*,#3927,.F.);
#5427=ORIENTED_EDGE('',*,*,#3855,.T.);
#5428=ORIENTED_EDGE('',*,*,#3731,.F.);
#5429=ORIENTED_EDGE('',*,*,#3734,.T.);
#5430=ORIENTED_EDGE('',*,*,#3733,.F.);
#5431=ORIENTED_EDGE('',*,*,#3854,.T.);
#5432=ORIENTED_EDGE('',*,*,#3928,.F.);
#5433=ORIENTED_EDGE('',*,*,#3925,.T.);
#5434=ORIENTED_EDGE('',*,*,#3727,.F.);
#5435=ORIENTED_EDGE('',*,*,#3926,.T.);
#5436=ORIENTED_EDGE('',*,*,#3928,.T.);
#5437=ORIENTED_EDGE('',*,*,#3853,.T.);
#5438=ORIENTED_EDGE('',*,*,#3868,.F.);
#5439=ORIENTED_EDGE('',*,*,#3794,.T.);
#5440=ORIENTED_EDGE('',*,*,#3883,.T.);
#5441=ORIENTED_EDGE('',*,*,#3929,.F.);
#5442=ORIENTED_EDGE('',*,*,#3930,.F.);
#5443=ORIENTED_EDGE('',*,*,#3931,.F.);
#5444=ORIENTED_EDGE('',*,*,#3932,.F.);
#5445=ORIENTED_EDGE('',*,*,#3933,.F.);
#5446=ORIENTED_EDGE('',*,*,#3869,.T.);
#5447=ORIENTED_EDGE('',*,*,#3810,.T.);
#5448=ORIENTED_EDGE('',*,*,#3822,.T.);
#5449=ORIENTED_EDGE('',*,*,#3929,.T.);
#5450=ORIENTED_EDGE('',*,*,#3882,.F.);
#5451=ORIENTED_EDGE('',*,*,#3934,.T.);
#5452=ORIENTED_EDGE('',*,*,#3935,.T.);
#5453=ORIENTED_EDGE('',*,*,#3930,.T.);
#5454=ORIENTED_EDGE('',*,*,#3935,.F.);
#5455=ORIENTED_EDGE('',*,*,#3936,.F.);
#5456=ORIENTED_EDGE('',*,*,#3937,.F.);
#5457=ORIENTED_EDGE('',*,*,#3931,.T.);
#5458=ORIENTED_EDGE('',*,*,#3937,.T.);
#5459=ORIENTED_EDGE('',*,*,#3938,.T.);
#5460=ORIENTED_EDGE('',*,*,#3939,.T.);
#5461=ORIENTED_EDGE('',*,*,#3933,.T.);
#5462=ORIENTED_EDGE('',*,*,#3940,.T.);
#5463=ORIENTED_EDGE('',*,*,#3941,.T.);
#5464=ORIENTED_EDGE('',*,*,#3870,.F.);
#5465=ORIENTED_EDGE('',*,*,#3932,.T.);
#5466=ORIENTED_EDGE('',*,*,#3939,.F.);
#5467=ORIENTED_EDGE('',*,*,#3942,.F.);
#5468=ORIENTED_EDGE('',*,*,#3940,.F.);
#5469=ORIENTED_EDGE('',*,*,#3943,.T.);
#5470=ORIENTED_EDGE('',*,*,#3944,.T.);
#5471=ORIENTED_EDGE('',*,*,#3942,.T.);
#5472=ORIENTED_EDGE('',*,*,#3945,.T.);
#5473=ORIENTED_EDGE('',*,*,#3946,.T.);
#5474=ORIENTED_EDGE('',*,*,#3947,.T.);
#5475=ORIENTED_EDGE('',*,*,#3936,.T.);
#5476=ORIENTED_EDGE('',*,*,#3948,.T.);
#5477=ORIENTED_EDGE('',*,*,#3949,.T.);
#5478=ORIENTED_EDGE('',*,*,#3943,.F.);
#5479=ORIENTED_EDGE('',*,*,#3938,.F.);
#5480=ORIENTED_EDGE('',*,*,#3949,.F.);
#5481=ORIENTED_EDGE('',*,*,#3860,.F.);
#5482=ORIENTED_EDGE('',*,*,#3881,.F.);
#5483=ORIENTED_EDGE('',*,*,#3861,.F.);
#5484=ORIENTED_EDGE('',*,*,#3948,.F.);
#5485=ORIENTED_EDGE('',*,*,#3934,.F.);
#5486=ORIENTED_EDGE('',*,*,#3950,.T.);
#5487=ORIENTED_EDGE('',*,*,#3907,.T.);
#5488=ORIENTED_EDGE('',*,*,#3951,.T.);
#5489=ORIENTED_EDGE('',*,*,#3951,.F.);
#5490=ORIENTED_EDGE('',*,*,#3910,.F.);
#5491=ORIENTED_EDGE('',*,*,#3947,.F.);
#5492=ORIENTED_EDGE('',*,*,#3952,.F.);
#5493=ORIENTED_EDGE('',*,*,#3889,.F.);
#5494=ORIENTED_EDGE('',*,*,#3904,.F.);
#5495=ORIENTED_EDGE('',*,*,#3950,.F.);
#5496=ORIENTED_EDGE('',*,*,#3953,.F.);
#5497=ORIENTED_EDGE('',*,*,#3891,.F.);
#5498=ORIENTED_EDGE('',*,*,#3954,.F.);
#5499=ORIENTED_EDGE('',*,*,#3946,.F.);
#5500=ORIENTED_EDGE('',*,*,#3912,.F.);
#5501=ORIENTED_EDGE('',*,*,#3899,.T.);
#5502=ORIENTED_EDGE('',*,*,#3913,.F.);
#5503=ORIENTED_EDGE('',*,*,#3945,.F.);
#5504=ORIENTED_EDGE('',*,*,#3909,.F.);
#5505=ORIENTED_EDGE('',*,*,#3871,.F.);
#5506=ORIENTED_EDGE('',*,*,#3941,.F.);
#5507=ORIENTED_EDGE('',*,*,#3944,.F.);
#5508=ORIENTED_EDGE('',*,*,#3859,.F.);
#5509=ORIENTED_EDGE('',*,*,#3953,.T.);
#5510=ORIENTED_EDGE('',*,*,#3952,.T.);
#5511=ORIENTED_EDGE('',*,*,#3954,.T.);
#5512=ORIENTED_EDGE('',*,*,#3890,.F.);
#5513=ORIENTED_EDGE('',*,*,#3955,.F.);
#5514=ORIENTED_EDGE('',*,*,#3956,.F.);
#5515=ORIENTED_EDGE('',*,*,#3957,.F.);
#5516=ORIENTED_EDGE('',*,*,#3958,.F.);
#5517=ORIENTED_EDGE('',*,*,#3959,.F.);
#5518=ORIENTED_EDGE('',*,*,#3960,.F.);
#5519=ORIENTED_EDGE('',*,*,#3961,.F.);
#5520=ORIENTED_EDGE('',*,*,#3962,.F.);
#5521=ORIENTED_EDGE('',*,*,#3963,.F.);
#5522=ORIENTED_EDGE('',*,*,#3955,.T.);
#5523=ORIENTED_EDGE('',*,*,#3964,.T.);
#5524=ORIENTED_EDGE('',*,*,#3962,.T.);
#5525=ORIENTED_EDGE('',*,*,#3965,.T.);
#5526=ORIENTED_EDGE('',*,*,#3879,.T.);
#5527=ORIENTED_EDGE('',*,*,#3966,.T.);
#5528=ORIENTED_EDGE('',*,*,#3963,.T.);
#5529=ORIENTED_EDGE('',*,*,#3967,.T.);
#5530=ORIENTED_EDGE('',*,*,#3968,.F.);
#5531=ORIENTED_EDGE('',*,*,#3969,.F.);
#5532=ORIENTED_EDGE('',*,*,#3970,.F.);
#5533=ORIENTED_EDGE('',*,*,#3969,.T.);
#5534=ORIENTED_EDGE('',*,*,#3971,.T.);
#5535=ORIENTED_EDGE('',*,*,#3959,.T.);
#5536=ORIENTED_EDGE('',*,*,#3972,.T.);
#5537=ORIENTED_EDGE('',*,*,#3961,.T.);
#5538=ORIENTED_EDGE('',*,*,#3973,.T.);
#5539=ORIENTED_EDGE('',*,*,#3970,.T.);
#5540=ORIENTED_EDGE('',*,*,#3974,.T.);
#5541=ORIENTED_EDGE('',*,*,#3877,.T.);
#5542=ORIENTED_EDGE('',*,*,#3975,.T.);
#5543=ORIENTED_EDGE('',*,*,#3968,.T.);
#5544=ORIENTED_EDGE('',*,*,#3976,.T.);
#5545=ORIENTED_EDGE('',*,*,#3875,.T.);
#5546=ORIENTED_EDGE('',*,*,#3977,.T.);
#5547=ORIENTED_EDGE('',*,*,#3960,.T.);
#5548=ORIENTED_EDGE('',*,*,#3978,.T.);
#5549=ORIENTED_EDGE('',*,*,#3958,.T.);
#5550=ORIENTED_EDGE('',*,*,#3979,.T.);
#5551=ORIENTED_EDGE('',*,*,#3956,.T.);
#5552=ORIENTED_EDGE('',*,*,#3980,.T.);
#5553=ORIENTED_EDGE('',*,*,#3873,.T.);
#5554=ORIENTED_EDGE('',*,*,#3981,.T.);
#5555=ORIENTED_EDGE('',*,*,#3957,.T.);
#5556=ORIENTED_EDGE('',*,*,#3982,.T.);
#5557=ORIENTED_EDGE('',*,*,#3976,.F.);
#5558=ORIENTED_EDGE('',*,*,#3973,.F.);
#5559=ORIENTED_EDGE('',*,*,#3966,.F.);
#5560=ORIENTED_EDGE('',*,*,#3878,.F.);
#5561=ORIENTED_EDGE('',*,*,#3792,.T.);
#5562=ORIENTED_EDGE('',*,*,#3880,.F.);
#5563=ORIENTED_EDGE('',*,*,#3967,.F.);
#5564=ORIENTED_EDGE('',*,*,#3964,.F.);
#5565=ORIENTED_EDGE('',*,*,#3981,.F.);
#5566=ORIENTED_EDGE('',*,*,#3872,.F.);
#5567=ORIENTED_EDGE('',*,*,#3808,.T.);
#5568=ORIENTED_EDGE('',*,*,#3821,.T.);
#5569=ORIENTED_EDGE('',*,*,#3972,.F.);
#5570=ORIENTED_EDGE('',*,*,#3980,.F.);
#5571=ORIENTED_EDGE('',*,*,#3965,.F.);
#5572=ORIENTED_EDGE('',*,*,#3974,.F.);
#5573=ORIENTED_EDGE('',*,*,#3767,.T.);
#5574=ORIENTED_EDGE('',*,*,#3783,.T.);
#5575=ORIENTED_EDGE('',*,*,#3780,.T.);
#5576=ORIENTED_EDGE('',*,*,#3777,.T.);
#5577=ORIENTED_EDGE('',*,*,#3774,.T.);
#5578=ORIENTED_EDGE('',*,*,#3771,.T.);
#5579=ORIENTED_EDGE('',*,*,#3748,.T.);
#5580=ORIENTED_EDGE('',*,*,#3764,.T.);
#5581=ORIENTED_EDGE('',*,*,#3761,.T.);
#5582=ORIENTED_EDGE('',*,*,#3758,.T.);
#5583=ORIENTED_EDGE('',*,*,#3755,.T.);
#5584=ORIENTED_EDGE('',*,*,#3752,.T.);
#5585=ORIENTED_EDGE('',*,*,#3745,.T.);
#5586=ORIENTED_EDGE('',*,*,#3743,.T.);
#5587=ORIENTED_EDGE('',*,*,#3741,.T.);
#5588=ORIENTED_EDGE('',*,*,#3738,.T.);
#5589=ORIENTED_EDGE('',*,*,#3977,.F.);
#5590=ORIENTED_EDGE('',*,*,#3874,.F.);
#5591=ORIENTED_EDGE('',*,*,#3982,.F.);
#5592=ORIENTED_EDGE('',*,*,#3979,.F.);
#5593=ORIENTED_EDGE('',*,*,#3975,.F.);
#5594=ORIENTED_EDGE('',*,*,#3876,.F.);
#5595=ORIENTED_EDGE('',*,*,#3978,.F.);
#5596=ORIENTED_EDGE('',*,*,#3971,.F.);
#6331=CYLINDRICAL_SURFACE('',#7148,0.15);
#6332=CYLINDRICAL_SURFACE('',#7151,0.15);
#6333=CYLINDRICAL_SURFACE('',#7153,0.15);
#6334=CYLINDRICAL_SURFACE('',#7155,0.15);
#6335=CYLINDRICAL_SURFACE('',#7174,0.17);
#6336=CYLINDRICAL_SURFACE('',#7176,0.17);
#6337=CYLINDRICAL_SURFACE('',#7200,0.4);
#6338=CYLINDRICAL_SURFACE('',#7202,0.4);
#6339=CYLINDRICAL_SURFACE('',#7224,0.1);
#6340=CYLINDRICAL_SURFACE('',#7228,0.1);
#6341=CYLINDRICAL_SURFACE('',#7242,0.3);
#6342=CYLINDRICAL_SURFACE('',#7247,0.3);
#6583=ADVANCED_FACE('',(#964,#618,#619,#620),#734,.F.);
#6584=ADVANCED_FACE('',(#965),#6331,.F.);
#6585=ADVANCED_FACE('',(#966),#6332,.F.);
#6586=ADVANCED_FACE('',(#967),#6333,.F.);
#6587=ADVANCED_FACE('',(#968),#6334,.F.);
#6588=ADVANCED_FACE('',(#969),#735,.F.);
#6589=ADVANCED_FACE('',(#970),#736,.F.);
#6590=ADVANCED_FACE('',(#971),#737,.F.);
#6591=ADVANCED_FACE('',(#972),#738,.F.);
#6592=ADVANCED_FACE('',(#973),#739,.F.);
#6593=ADVANCED_FACE('',(#974),#740,.F.);
#6594=ADVANCED_FACE('',(#975,#621),#741,.F.);
#6595=ADVANCED_FACE('',(#976),#742,.F.);
#6596=ADVANCED_FACE('',(#977),#743,.F.);
#6597=ADVANCED_FACE('',(#978),#744,.F.);
#6598=ADVANCED_FACE('',(#979),#745,.F.);
#6599=ADVANCED_FACE('',(#980),#746,.F.);
#6600=ADVANCED_FACE('',(#981),#747,.F.);
#6601=ADVANCED_FACE('',(#982,#622),#748,.F.);
#6602=ADVANCED_FACE('',(#983),#6335,.F.);
#6603=ADVANCED_FACE('',(#984),#6336,.F.);
#6604=ADVANCED_FACE('',(#985),#749,.F.);
#6605=ADVANCED_FACE('',(#986),#750,.F.);
#6606=ADVANCED_FACE('',(#987),#751,.F.);
#6607=ADVANCED_FACE('',(#988),#752,.F.);
#6608=ADVANCED_FACE('',(#989),#753,.F.);
#6609=ADVANCED_FACE('',(#990),#754,.F.);
#6610=ADVANCED_FACE('',(#991),#755,.F.);
#6611=ADVANCED_FACE('',(#992,#623),#756,.F.);
#6612=ADVANCED_FACE('',(#993,#624),#757,.F.);
#6613=ADVANCED_FACE('',(#994),#758,.F.);
#6614=ADVANCED_FACE('',(#995),#759,.F.);
#6615=ADVANCED_FACE('',(#996),#760,.F.);
#6616=ADVANCED_FACE('',(#997),#761,.F.);
#6617=ADVANCED_FACE('',(#998),#762,.F.);
#6618=ADVANCED_FACE('',(#999),#763,.T.);
#6619=ADVANCED_FACE('',(#1000),#764,.T.);
#6620=ADVANCED_FACE('',(#1001),#765,.T.);
#6621=ADVANCED_FACE('',(#1002),#766,.T.);
#6622=ADVANCED_FACE('',(#1003),#767,.T.);
#6623=ADVANCED_FACE('',(#1004,#625),#768,.F.);
#6624=ADVANCED_FACE('',(#1005),#6337,.T.);
#6625=ADVANCED_FACE('',(#1006),#6338,.T.);
#6626=ADVANCED_FACE('',(#1007),#769,.T.);
#6627=ADVANCED_FACE('',(#1008),#124,.T.);
#6628=ADVANCED_FACE('',(#1009),#125,.T.);
#6629=ADVANCED_FACE('',(#1010),#126,.T.);
#6630=ADVANCED_FACE('',(#1011),#127,.T.);
#6631=ADVANCED_FACE('',(#1012,#626,#627,#628),#770,.F.);
#6632=ADVANCED_FACE('',(#1013),#771,.F.);
#6633=ADVANCED_FACE('',(#1014),#128,.T.);
#6634=ADVANCED_FACE('',(#1015),#129,.T.);
#6635=ADVANCED_FACE('',(#1016),#130,.T.);
#6636=ADVANCED_FACE('',(#1017),#772,.T.);
#6637=ADVANCED_FACE('',(#1018),#131,.T.);
#6638=ADVANCED_FACE('',(#1019),#132,.T.);
#6639=ADVANCED_FACE('',(#1020),#773,.F.);
#6640=ADVANCED_FACE('',(#1021),#133,.T.);
#6641=ADVANCED_FACE('',(#1022),#134,.T.);
#6642=ADVANCED_FACE('',(#1023),#774,.T.);
#6643=ADVANCED_FACE('',(#1024),#135,.T.);
#6644=ADVANCED_FACE('',(#1025),#136,.T.);
#6645=ADVANCED_FACE('',(#1026),#137,.T.);
#6646=ADVANCED_FACE('',(#1027),#138,.T.);
#6647=ADVANCED_FACE('',(#1028),#775,.T.);
#6648=ADVANCED_FACE('',(#1029),#139,.T.);
#6649=ADVANCED_FACE('',(#1030),#140,.T.);
#6650=ADVANCED_FACE('',(#1031),#776,.F.);
#6651=ADVANCED_FACE('',(#1032),#141,.T.);
#6652=ADVANCED_FACE('',(#1033),#142,.T.);
#6653=ADVANCED_FACE('',(#1034),#84,.F.);
#6654=ADVANCED_FACE('',(#1035),#85,.F.);
#6655=ADVANCED_FACE('',(#1036),#86,.F.);
#6656=ADVANCED_FACE('',(#1037),#6339,.F.);
#6657=ADVANCED_FACE('',(#1038),#143,.T.);
#6658=ADVANCED_FACE('',(#1039),#87,.F.);
#6659=ADVANCED_FACE('',(#1040),#6340,.F.);
#6660=ADVANCED_FACE('',(#1041),#144,.T.);
#6661=ADVANCED_FACE('',(#1042),#145,.T.);
#6662=ADVANCED_FACE('',(#1043),#146,.T.);
#6663=ADVANCED_FACE('',(#1044),#147,.T.);
#6664=ADVANCED_FACE('',(#1045),#777,.T.);
#6665=ADVANCED_FACE('',(#1046),#88,.T.);
#6666=ADVANCED_FACE('',(#1047),#89,.T.);
#6667=ADVANCED_FACE('',(#1048),#90,.T.);
#6668=ADVANCED_FACE('',(#1049),#6341,.T.);
#6669=ADVANCED_FACE('',(#1050),#148,.F.);
#6670=ADVANCED_FACE('',(#1051),#91,.T.);
#6671=ADVANCED_FACE('',(#1052),#6342,.T.);
#6672=ADVANCED_FACE('',(#1053),#149,.F.);
#6673=ADVANCED_FACE('',(#1054),#150,.F.);
#6674=ADVANCED_FACE('',(#1055),#151,.F.);
#6675=ADVANCED_FACE('',(#1056),#152,.F.);
#6676=ADVANCED_FACE('',(#1057),#153,.F.);
#6677=ADVANCED_FACE('',(#1058),#154,.F.);
#6678=ADVANCED_FACE('',(#1059),#778,.F.);
#6679=ADVANCED_FACE('',(#1060,#629,#630,#631,#632,#633,#634),#779,.T.);
#6680=ADVANCED_FACE('',(#1061),#155,.F.);
#6681=ADVANCED_FACE('',(#1062),#780,.F.);
#6825=CLOSED_SHELL('',(#6583,#6584,#6585,#6586,#6587,#6588,#6589,#6590,
#6591,#6592,#6593,#6594,#6595,#6596,#6597,#6598,#6599,#6600,#6601,#6602,
#6603,#6604,#6605,#6606,#6607,#6608,#6609,#6610,#6611,#6612,#6613,#6614,
#6615,#6616,#6617,#6618,#6619,#6620,#6621,#6622,#6623,#6624,#6625,#6626,
#6627,#6628,#6629,#6630,#6631,#6632,#6633,#6634,#6635,#6636,#6637,#6638,
#6639,#6640,#6641,#6642,#6643,#6644,#6645,#6646,#6647,#6648,#6649,#6650,
#6651,#6652,#6653,#6654,#6655,#6656,#6657,#6658,#6659,#6660,#6661,#6662,
#6663,#6664,#6665,#6666,#6667,#6668,#6669,#6670,#6671,#6672,#6673,#6674,
#6675,#6676,#6677,#6678,#6679,#6680,#6681));
#7143=AXIS2_PLACEMENT_3D('',#11241,#8044,#8045);
#7144=AXIS2_PLACEMENT_3D('',#11242,#8046,#8047);
#7145=AXIS2_PLACEMENT_3D('',#11308,#8050,#8051);
#7146=AXIS2_PLACEMENT_3D('',#11310,#8052,#8053);
#7147=AXIS2_PLACEMENT_3D('',#11312,#8054,#8055);
#7148=AXIS2_PLACEMENT_3D('',#11313,#8056,#8057);
#7149=AXIS2_PLACEMENT_3D('',#11315,#8058,#8059);
#7150=AXIS2_PLACEMENT_3D('',#11318,#8061,#8062);
#7151=AXIS2_PLACEMENT_3D('',#11319,#8063,#8064);
#7152=AXIS2_PLACEMENT_3D('',#11321,#8065,#8066);
#7153=AXIS2_PLACEMENT_3D('',#11323,#8068,#8069);
#7154=AXIS2_PLACEMENT_3D('',#11325,#8070,#8071);
#7155=AXIS2_PLACEMENT_3D('',#11327,#8073,#8074);
#7156=AXIS2_PLACEMENT_3D('',#11329,#8075,#8076);
#7157=AXIS2_PLACEMENT_3D('',#11332,#8078,#8079);
#7158=AXIS2_PLACEMENT_3D('',#11333,#8080,#8081);
#7159=AXIS2_PLACEMENT_3D('',#11342,#8086,#8087);
#7160=AXIS2_PLACEMENT_3D('',#11348,#8091,#8092);
#7161=AXIS2_PLACEMENT_3D('',#11354,#8096,#8097);
#7162=AXIS2_PLACEMENT_3D('',#11360,#8101,#8102);
#7163=AXIS2_PLACEMENT_3D('',#11366,#8106,#8107);
#7164=AXIS2_PLACEMENT_3D('',#11369,#8110,#8111);
#7165=AXIS2_PLACEMENT_3D('',#11371,#8112,#8113);
#7166=AXIS2_PLACEMENT_3D('',#11372,#8114,#8115);
#7167=AXIS2_PLACEMENT_3D('',#11381,#8120,#8121);
#7168=AXIS2_PLACEMENT_3D('',#11387,#8125,#8126);
#7169=AXIS2_PLACEMENT_3D('',#11393,#8130,#8131);
#7170=AXIS2_PLACEMENT_3D('',#11399,#8135,#8136);
#7171=AXIS2_PLACEMENT_3D('',#11405,#8140,#8141);
#7172=AXIS2_PLACEMENT_3D('',#11408,#8144,#8145);
#7173=AXIS2_PLACEMENT_3D('',#11410,#8146,#8147);
#7174=AXIS2_PLACEMENT_3D('',#11411,#8148,#8149);
#7175=AXIS2_PLACEMENT_3D('',#11414,#8151,#8152);
#7176=AXIS2_PLACEMENT_3D('',#11415,#8153,#8154);
#7177=AXIS2_PLACEMENT_3D('',#11418,#8156,#8157);
#7178=AXIS2_PLACEMENT_3D('',#11419,#8158,#8159);
#7179=AXIS2_PLACEMENT_3D('',#11428,#8164,#8165);
#7180=AXIS2_PLACEMENT_3D('',#11437,#8170,#8171);
#7181=AXIS2_PLACEMENT_3D('',#11446,#8176,#8177);
#7182=AXIS2_PLACEMENT_3D('',#11455,#8182,#8183);
#7183=AXIS2_PLACEMENT_3D('',#11464,#8188,#8189);
#7184=AXIS2_PLACEMENT_3D('',#11473,#8194,#8195);
#7185=AXIS2_PLACEMENT_3D('',#11482,#8200,#8201);
#7186=AXIS2_PLACEMENT_3D('',#11484,#8202,#8203);
#7187=AXIS2_PLACEMENT_3D('',#11485,#8204,#8205);
#7188=AXIS2_PLACEMENT_3D('',#11487,#8206,#8207);
#7189=AXIS2_PLACEMENT_3D('',#11488,#8208,#8209);
#7190=AXIS2_PLACEMENT_3D('',#11491,#8212,#8213);
#7191=AXIS2_PLACEMENT_3D('',#11494,#8216,#8217);
#7192=AXIS2_PLACEMENT_3D('',#11497,#8220,#8221);
#7193=AXIS2_PLACEMENT_3D('',#11503,#8225,#8226);
#7194=AXIS2_PLACEMENT_3D('',#11509,#8230,#8231);
#7195=AXIS2_PLACEMENT_3D('',#11586,#8234,#8235);
#7196=AXIS2_PLACEMENT_3D('',#11664,#8239,#8240);
#7197=AXIS2_PLACEMENT_3D('',#11742,#8244,#8245);
#7198=AXIS2_PLACEMENT_3D('',#11817,#8248,#8249);
#7199=AXIS2_PLACEMENT_3D('',#11833,#8253,#8254);
#7200=AXIS2_PLACEMENT_3D('',#12211,#8266,#8267);
#7201=AXIS2_PLACEMENT_3D('',#12213,#8268,#8269);
#7202=AXIS2_PLACEMENT_3D('',#12215,#8271,#8272);
#7203=AXIS2_PLACEMENT_3D('',#12217,#8274,#8275);
#7204=AXIS2_PLACEMENT_3D('',#12385,#8277,#8278);
#7205=AXIS2_PLACEMENT_3D('',#12386,#8279,#8280);
#7206=AXIS2_PLACEMENT_3D('',#12391,#8281,#8282);
#7207=AXIS2_PLACEMENT_3D('',#12463,#8284,#8285);
#7208=AXIS2_PLACEMENT_3D('',#12581,#8287,#8288);
#7209=AXIS2_PLACEMENT_3D('',#12626,#8289,#8290);
#7210=AXIS2_PLACEMENT_3D('',#12777,#8291,#8292);
#7211=AXIS2_PLACEMENT_3D('',#12897,#8294,#8295);
#7212=AXIS2_PLACEMENT_3D('',#12902,#8296,#8297);
#7213=AXIS2_PLACEMENT_3D('',#12954,#8299,#8300);
#7214=AXIS2_PLACEMENT_3D('',#12955,#8301,#8302);
#7215=AXIS2_PLACEMENT_3D('',#12956,#8303,#8304);
#7216=AXIS2_PLACEMENT_3D('',#12957,#8305,#8306);
#7217=AXIS2_PLACEMENT_3D('',#12958,#8307,#8308);
#7218=AXIS2_PLACEMENT_3D('',#12959,#8309,#8310);
#7219=AXIS2_PLACEMENT_3D('',#12961,#8311,#8312);
#7220=AXIS2_PLACEMENT_3D('',#12962,#8313,#8314);
#7221=AXIS2_PLACEMENT_3D('',#12963,#8315,#8316);
#7222=AXIS2_PLACEMENT_3D('',#12964,#8317,#8318);
#7223=AXIS2_PLACEMENT_3D('',#12965,#8319,#8320);
#7224=AXIS2_PLACEMENT_3D('',#12966,#8321,#8322);
#7225=AXIS2_PLACEMENT_3D('',#12987,#8323,#8324);
#7226=AXIS2_PLACEMENT_3D('',#12989,#8325,#8326);
#7227=AXIS2_PLACEMENT_3D('',#12990,#8327,#8328);
#7228=AXIS2_PLACEMENT_3D('',#12991,#8329,#8330);
#7229=AXIS2_PLACEMENT_3D('',#13089,#8332,#8333);
#7230=AXIS2_PLACEMENT_3D('',#13090,#8334,#8335);
#7231=AXIS2_PLACEMENT_3D('',#13093,#8336,#8337);
#7232=AXIS2_PLACEMENT_3D('',#13095,#8338,#8339);
#7233=AXIS2_PLACEMENT_3D('',#13096,#8340,#8341);
#7234=AXIS2_PLACEMENT_3D('',#13097,#8342,#8343);
#7235=AXIS2_PLACEMENT_3D('',#13100,#8344,#8345);
#7236=AXIS2_PLACEMENT_3D('',#13102,#8346,#8347);
#7237=AXIS2_PLACEMENT_3D('',#13103,#8348,#8349);
#7238=AXIS2_PLACEMENT_3D('',#13104,#8350,#8351);
#7239=AXIS2_PLACEMENT_3D('',#13107,#8352,#8353);
#7240=AXIS2_PLACEMENT_3D('',#13109,#8354,#8355);
#7241=AXIS2_PLACEMENT_3D('',#13110,#8356,#8357);
#7242=AXIS2_PLACEMENT_3D('',#13111,#8358,#8359);
#7243=AXIS2_PLACEMENT_3D('',#13142,#8362,#8363);
#7244=AXIS2_PLACEMENT_3D('',#13145,#8364,#8365);
#7245=AXIS2_PLACEMENT_3D('',#13147,#8366,#8367);
#7246=AXIS2_PLACEMENT_3D('',#13148,#8368,#8369);
#7247=AXIS2_PLACEMENT_3D('',#13149,#8370,#8371);
#7248=AXIS2_PLACEMENT_3D('',#13330,#8374,#8375);
#7249=AXIS2_PLACEMENT_3D('',#13331,#8376,#8377);
#7250=AXIS2_PLACEMENT_3D('',#13348,#8378,#8379);
#8044=DIRECTION('axis',(0.,0.,1.));
#8045=DIRECTION('refdir',(1.,0.,0.));
#8046=DIRECTION('center_axis',(-9.61618982193066E-33,1.03600583455278E-18,
1.));
#8047=DIRECTION('ref_axis',(1.,0.,9.61618982193066E-33));
#8048=DIRECTION('',(0.,-1.,1.03600583455278E-18));
#8049=DIRECTION('',(0.,1.,-1.03600583455278E-18));
#8050=DIRECTION('center_axis',(-9.61618982193066E-33,1.03600583455278E-18,
1.));
#8051=DIRECTION('ref_axis',(1.,0.,0.));
#8052=DIRECTION('center_axis',(-9.61618982193066E-33,1.03600583455278E-18,
1.));
#8053=DIRECTION('ref_axis',(1.,0.,0.));
#8054=DIRECTION('center_axis',(-9.61618982193066E-33,1.03600583455278E-18,
1.));
#8055=DIRECTION('ref_axis',(1.,0.,0.));
#8056=DIRECTION('center_axis',(0.,0.,-1.));
#8057=DIRECTION('ref_axis',(1.,0.,0.));
#8058=DIRECTION('center_axis',(9.61618982193066E-33,-1.03600583455278E-18,
-1.));
#8059=DIRECTION('ref_axis',(1.,0.,0.));
#8060=DIRECTION('',(0.,0.,-1.));
#8061=DIRECTION('center_axis',(-9.61618982193066E-33,1.03600583455278E-18,
1.));
#8062=DIRECTION('ref_axis',(1.,0.,0.));
#8063=DIRECTION('center_axis',(0.,0.,-1.));
#8064=DIRECTION('ref_axis',(1.,0.,0.));
#8065=DIRECTION('center_axis',(9.61618982193066E-33,-1.03600583455278E-18,
-1.));
#8066=DIRECTION('ref_axis',(1.,0.,0.));
#8067=DIRECTION('',(0.,0.,-1.));
#8068=DIRECTION('center_axis',(0.,0.,-1.));
#8069=DIRECTION('ref_axis',(1.,0.,0.));
#8070=DIRECTION('center_axis',(9.61618982193066E-33,-1.03600583455278E-18,
-1.));
#8071=DIRECTION('ref_axis',(1.,0.,0.));
#8072=DIRECTION('',(0.,0.,-1.));
#8073=DIRECTION('center_axis',(0.,0.,-1.));
#8074=DIRECTION('ref_axis',(1.,0.,0.));
#8075=DIRECTION('center_axis',(9.61618982193066E-33,-1.03600583455278E-18,
-1.));
#8076=DIRECTION('ref_axis',(1.,0.,0.));
#8077=DIRECTION('',(0.,0.,-1.));
#8078=DIRECTION('center_axis',(-9.61618982193066E-33,1.03600583455278E-18,
1.));
#8079=DIRECTION('ref_axis',(1.,0.,0.));
#8080=DIRECTION('center_axis',(0.86602540378444,0.499999999999998,0.));
#8081=DIRECTION('ref_axis',(0.499999999999998,-0.86602540378444,0.));
#8082=DIRECTION('',(0.499999999999998,-0.86602540378444,8.9720737119161E-19));
#8083=DIRECTION('',(0.,0.,-1.));
#8084=DIRECTION('',(0.499999999999998,-0.86602540378444,0.));
#8085=DIRECTION('',(0.,0.,-1.));
#8086=DIRECTION('center_axis',(1.60246890531964E-16,1.,0.));
#8087=DIRECTION('ref_axis',(1.,-1.60246890531964E-16,0.));
#8088=DIRECTION('',(1.,-1.60246890531964E-16,9.78220653549071E-33));
#8089=DIRECTION('',(0.,0.,-1.));
#8090=DIRECTION('',(1.,-1.60246890531964E-16,0.));
#8091=DIRECTION('center_axis',(-0.86602540378444,0.499999999999998,0.));
#8092=DIRECTION('ref_axis',(0.499999999999998,0.86602540378444,0.));
#8093=DIRECTION('',(0.499999999999998,0.86602540378444,-8.97207371191601E-19));
#8094=DIRECTION('',(0.,0.,-1.));
#8095=DIRECTION('',(0.499999999999998,0.86602540378444,0.));
#8096=DIRECTION('center_axis',(-0.86602540378444,-0.499999999999998,0.));
#8097=DIRECTION('ref_axis',(-0.499999999999998,0.86602540378444,0.));
#8098=DIRECTION('',(-0.499999999999998,0.86602540378444,-8.9720737119161E-19));
#8099=DIRECTION('',(0.,0.,-1.));
#8100=DIRECTION('',(-0.499999999999998,0.86602540378444,0.));
#8101=DIRECTION('center_axis',(-1.60246890531964E-16,-1.,0.));
#8102=DIRECTION('ref_axis',(-1.,1.60246890531964E-16,0.));
#8103=DIRECTION('',(-1.,1.60246890531964E-16,-9.78220653549071E-33));
#8104=DIRECTION('',(0.,0.,-1.));
#8105=DIRECTION('',(-1.,1.60246890531964E-16,0.));
#8106=DIRECTION('center_axis',(0.86602540378444,-0.499999999999998,0.));
#8107=DIRECTION('ref_axis',(-0.499999999999998,-0.86602540378444,0.));
#8108=DIRECTION('',(-0.499999999999998,-0.86602540378444,8.97207371191601E-19));
#8109=DIRECTION('',(-0.499999999999998,-0.86602540378444,0.));
#8110=DIRECTION('center_axis',(0.,0.,-1.));
#8111=DIRECTION('ref_axis',(-1.,0.,0.));
#8112=DIRECTION('center_axis',(0.,0.,1.));
#8113=DIRECTION('ref_axis',(1.,0.,0.));
#8114=DIRECTION('center_axis',(0.866025403784439,0.5,0.));
#8115=DIRECTION('ref_axis',(0.5,-0.866025403784439,0.));
#8116=DIRECTION('',(0.5,-0.866025403784439,8.97207371191609E-19));
#8117=DIRECTION('',(0.,0.,-1.));
#8118=DIRECTION('',(0.5,-0.866025403784439,0.));
#8119=DIRECTION('',(0.,0.,-1.));
#8120=DIRECTION('center_axis',(1.60246890531964E-16,1.,0.));
#8121=DIRECTION('ref_axis',(1.,-1.60246890531964E-16,0.));
#8122=DIRECTION('',(1.,-1.60246890531964E-16,9.78220653549071E-33));
#8123=DIRECTION('',(0.,0.,-1.));
#8124=DIRECTION('',(1.,-1.60246890531964E-16,0.));
#8125=DIRECTION('center_axis',(-0.866025403784438,0.5,0.));
#8126=DIRECTION('ref_axis',(0.5,0.866025403784438,0.));
#8127=DIRECTION('',(0.5,0.866025403784438,-8.97207371191599E-19));
#8128=DIRECTION('',(0.,0.,-1.));
#8129=DIRECTION('',(0.5,0.866025403784438,0.));
#8130=DIRECTION('center_axis',(-0.866025403784439,-0.499999999999999,0.));
#8131=DIRECTION('ref_axis',(-0.499999999999999,0.866025403784439,0.));
#8132=DIRECTION('',(-0.499999999999999,0.866025403784439,-8.97207371191609E-19));
#8133=DIRECTION('',(0.,0.,-1.));
#8134=DIRECTION('',(-0.499999999999999,0.866025403784439,0.));
#8135=DIRECTION('center_axis',(-1.60246890531964E-16,-1.,0.));
#8136=DIRECTION('ref_axis',(-1.,1.60246890531964E-16,0.));
#8137=DIRECTION('',(-1.,1.60246890531964E-16,-9.78220653549071E-33));
#8138=DIRECTION('',(0.,0.,-1.));
#8139=DIRECTION('',(-1.,1.60246890531964E-16,0.));
#8140=DIRECTION('center_axis',(0.866025403784439,-0.5,0.));
#8141=DIRECTION('ref_axis',(-0.5,-0.866025403784439,0.));
#8142=DIRECTION('',(-0.5,-0.866025403784439,8.97207371191599E-19));
#8143=DIRECTION('',(-0.5,-0.866025403784439,0.));
#8144=DIRECTION('center_axis',(0.,0.,-1.));
#8145=DIRECTION('ref_axis',(-1.,0.,0.));
#8146=DIRECTION('center_axis',(0.,0.,1.));
#8147=DIRECTION('ref_axis',(1.,0.,0.));
#8148=DIRECTION('center_axis',(0.,0.,-1.));
#8149=DIRECTION('ref_axis',(1.,0.,0.));
#8150=DIRECTION('',(0.,0.,-1.));
#8151=DIRECTION('center_axis',(0.,0.,1.));
#8152=DIRECTION('ref_axis',(1.,0.,0.));
#8153=DIRECTION('center_axis',(0.,0.,-1.));
#8154=DIRECTION('ref_axis',(1.,0.,0.));
#8155=DIRECTION('',(0.,0.,-1.));
#8156=DIRECTION('center_axis',(0.,0.,1.));
#8157=DIRECTION('ref_axis',(1.,0.,0.));
#8158=DIRECTION('center_axis',(0.,-1.,0.));
#8159=DIRECTION('ref_axis',(-1.,0.,0.));
#8160=DIRECTION('',(0.0523359562429438,0.,0.998629534754574));
#8161=DIRECTION('',(1.,0.,0.));
#8162=DIRECTION('',(-0.0523359562429438,0.,-0.998629534754574));
#8163=DIRECTION('',(1.,0.,0.));
#8164=DIRECTION('center_axis',(0.,-1.,0.));
#8165=DIRECTION('ref_axis',(-1.,0.,0.));
#8166=DIRECTION('',(0.,0.,-1.));
#8167=DIRECTION('',(1.,0.,0.));
#8168=DIRECTION('',(0.,0.,1.));
#8169=DIRECTION('',(1.,0.,0.));
#8170=DIRECTION('center_axis',(0.,-1.,0.));
#8171=DIRECTION('ref_axis',(-1.,0.,0.));
#8172=DIRECTION('',(0.,0.,-1.));
#8173=DIRECTION('',(1.,0.,0.));
#8174=DIRECTION('',(0.,0.,1.));
#8175=DIRECTION('',(1.,0.,0.));
#8176=DIRECTION('center_axis',(0.,-1.,0.));
#8177=DIRECTION('ref_axis',(-1.,0.,0.));
#8178=DIRECTION('',(0.,0.,-1.));
#8179=DIRECTION('',(1.,0.,0.));
#8180=DIRECTION('',(0.,0.,1.));
#8181=DIRECTION('',(1.,0.,0.));
#8182=DIRECTION('center_axis',(0.,1.,0.));
#8183=DIRECTION('ref_axis',(1.,0.,0.));
#8184=DIRECTION('',(-0.0523359562429438,0.,-0.998629534754574));
#8185=DIRECTION('',(-1.,0.,0.));
#8186=DIRECTION('',(0.0523359562429438,0.,0.998629534754574));
#8187=DIRECTION('',(-1.,0.,0.));
#8188=DIRECTION('center_axis',(0.,1.,0.));
#8189=DIRECTION('ref_axis',(1.,0.,0.));
#8190=DIRECTION('',(0.,0.,1.));
#8191=DIRECTION('',(-1.,0.,0.));
#8192=DIRECTION('',(0.,0.,-1.));
#8193=DIRECTION('',(-1.,0.,0.));
#8194=DIRECTION('center_axis',(0.,1.,0.));
#8195=DIRECTION('ref_axis',(1.,0.,0.));
#8196=DIRECTION('',(0.,0.,1.));
#8197=DIRECTION('',(-1.,0.,0.));
#8198=DIRECTION('',(0.,0.,-1.));
#8199=DIRECTION('',(-1.,0.,0.));
#8200=DIRECTION('center_axis',(0.,0.,1.));
#8201=DIRECTION('ref_axis',(1.,0.,0.));
#8202=DIRECTION('center_axis',(0.,0.,1.));
#8203=DIRECTION('ref_axis',(1.,0.,0.));
#8204=DIRECTION('center_axis',(0.,0.,1.));
#8205=DIRECTION('ref_axis',(1.,0.,0.));
#8206=DIRECTION('center_axis',(0.,0.,1.));
#8207=DIRECTION('ref_axis',(1.,0.,0.));
#8208=DIRECTION('center_axis',(0.,0.,1.));
#8209=DIRECTION('ref_axis',(1.,0.,0.));
#8210=DIRECTION('',(0.,1.,0.));
#8211=DIRECTION('',(0.,-1.,0.));
#8212=DIRECTION('center_axis',(0.,0.,1.));
#8213=DIRECTION('ref_axis',(1.,0.,0.));
#8214=DIRECTION('',(0.,-1.,0.));
#8215=DIRECTION('',(0.,1.,0.));
#8216=DIRECTION('center_axis',(0.,0.,1.));
#8217=DIRECTION('ref_axis',(1.,0.,0.));
#8218=DIRECTION('',(0.,-1.,0.));
#8219=DIRECTION('',(0.,1.,0.));
#8220=DIRECTION('center_axis',(0.,0.,1.));
#8221=DIRECTION('ref_axis',(1.,0.,0.));
#8222=DIRECTION('',(0.,-1.,0.));
#8223=DIRECTION('',(-1.,0.,0.));
#8224=DIRECTION('',(0.,1.,0.));
#8225=DIRECTION('center_axis',(0.,1.,0.));
#8226=DIRECTION('ref_axis',(1.,0.,0.));
#8227=DIRECTION('',(0.,0.,1.));
#8228=DIRECTION('',(-1.,0.,0.));
#8229=DIRECTION('',(0.,0.,-1.));
#8230=DIRECTION('center_axis',(-1.,0.,0.));
#8231=DIRECTION('ref_axis',(0.,-1.,0.));
#8232=DIRECTION('',(0.,-1.,0.));
#8233=DIRECTION('',(0.,-1.,1.03600583455278E-18));
#8234=DIRECTION('center_axis',(1.,0.,0.));
#8235=DIRECTION('ref_axis',(0.,1.,0.));
#8236=DIRECTION('',(0.,1.,0.));
#8237=DIRECTION('',(0.,1.,-1.03600583455278E-18));
#8238=DIRECTION('',(0.,1.,0.));
#8239=DIRECTION('center_axis',(1.,0.,0.));
#8240=DIRECTION('ref_axis',(0.,1.,0.));
#8241=DIRECTION('',(0.,1.,0.));
#8242=DIRECTION('',(0.,1.,-1.03600583455278E-18));
#8243=DIRECTION('',(0.,1.,0.));
#8244=DIRECTION('center_axis',(1.,0.,0.));
#8245=DIRECTION('ref_axis',(0.,1.,0.));
#8246=DIRECTION('',(0.,1.,0.));
#8247=DIRECTION('',(0.,1.,0.));
#8248=DIRECTION('center_axis',(0.998629534754574,0.,-0.0523359562429438));
#8249=DIRECTION('ref_axis',(-0.0523359562429438,0.,-0.998629534754574));
#8250=DIRECTION('',(0.,-1.,0.));
#8251=DIRECTION('',(5.42947651131849E-20,-1.,1.03600583455278E-18));
#8252=DIRECTION('',(0.,-1.,0.));
#8253=DIRECTION('center_axis',(0.,0.,1.));
#8254=DIRECTION('ref_axis',(1.,0.,0.));
#8255=DIRECTION('',(0.,-1.,0.));
#8256=DIRECTION('',(0.,-1.,0.));
#8257=DIRECTION('',(0.,-1.,0.));
#8258=DIRECTION('',(0.,1.,0.));
#8259=DIRECTION('',(0.,-1.,0.));
#8260=DIRECTION('',(0.,1.,0.));
#8261=DIRECTION('',(0.,-1.,0.));
#8262=DIRECTION('',(0.,-1.,0.));
#8263=DIRECTION('',(0.,-1.,0.));
#8264=DIRECTION('',(0.,1.,0.));
#8265=DIRECTION('',(0.,1.,0.));
#8266=DIRECTION('center_axis',(0.,0.,1.));
#8267=DIRECTION('ref_axis',(1.,0.,0.));
#8268=DIRECTION('center_axis',(-9.61618982193066E-33,1.03600583455278E-18,
1.));
#8269=DIRECTION('ref_axis',(1.,0.,0.));
#8270=DIRECTION('',(0.,0.,-1.));
#8271=DIRECTION('center_axis',(0.,0.,1.));
#8272=DIRECTION('ref_axis',(1.,0.,0.));
#8273=DIRECTION('',(0.,0.,-1.));
#8274=DIRECTION('center_axis',(1.,0.,0.));
#8275=DIRECTION('ref_axis',(0.,1.,0.));
#8276=DIRECTION('',(0.,1.,-1.03600583455278E-18));
#8277=DIRECTION('center_axis',(0.994044372876412,-0.108976074221552,-1.1933167131821E-14));
#8278=DIRECTION('ref_axis',(-0.108857570442347,-0.992963419871597,0.0466226999892957));
#8279=DIRECTION('center_axis',(-9.61618982193066E-33,1.03600583455278E-18,
1.));
#8280=DIRECTION('ref_axis',(1.,0.,9.61618982193066E-33));
#8281=DIRECTION('center_axis',(-9.61618982193066E-33,1.03600583455278E-18,
1.));
#8282=DIRECTION('ref_axis',(1.,0.,9.61618982193066E-33));
#8283=DIRECTION('',(-5.42947651131849E-20,-1.,1.03600583455278E-18));
#8284=DIRECTION('center_axis',(-1.,0.,0.));
#8285=DIRECTION('ref_axis',(0.,-1.,0.));
#8286=DIRECTION('',(0.,-1.,1.03600583455278E-18));
#8287=DIRECTION('center_axis',(-9.61618982193066E-33,1.03600583455278E-18,
1.));
#8288=DIRECTION('ref_axis',(1.,0.,9.61618982193066E-33));
#8289=DIRECTION('center_axis',(-1.,0.,0.));
#8290=DIRECTION('ref_axis',(0.,-1.,0.));
#8291=DIRECTION('center_axis',(-1.,0.,0.));
#8292=DIRECTION('ref_axis',(0.,-1.,0.));
#8293=DIRECTION('',(0.,-1.,1.03600583455278E-18));
#8294=DIRECTION('center_axis',(-0.999738255753194,0.0228783737088345,0.));
#8295=DIRECTION('ref_axis',(0.,0.,1.));
#8296=DIRECTION('center_axis',(-9.61618982193066E-33,1.03600583455278E-18,
1.));
#8297=DIRECTION('ref_axis',(1.,0.,9.61618982193066E-33));
#8298=DIRECTION('',(-5.42947651131849E-20,1.,-1.03600583455278E-18));
#8299=DIRECTION('center_axis',(-0.999738255790058,-0.0228783720979604,1.69987959829136E-9));
#8300=DIRECTION('ref_axis',(-0.022845652001536,0.998308458201847,0.0534630570326489));
#8301=DIRECTION('center_axis',(-0.375013085256251,-0.833398400631247,0.405970801550885));
#8302=DIRECTION('ref_axis',(-0.565498005067694,0.552672693214782,0.612180447612612));
#8303=DIRECTION('center_axis',(-7.78474640228738E-11,1.,0.));
#8304=DIRECTION('ref_axis',(0.,0.,1.));
#8305=DIRECTION('center_axis',(0.0522645732252412,-0.0522112666801462,0.997267465636596));
#8306=DIRECTION('ref_axis',(-0.998629534754574,0.,0.0523359562429445));
#8307=DIRECTION('center_axis',(0.361627795167438,-0.818371417997736,0.44664701943113));
#8308=DIRECTION('ref_axis',(0.514966362801186,0.574689674697898,0.636035708886648));
#8309=DIRECTION('center_axis',(0.994044372876412,0.108976074221546,-5.96658356591051E-15));
#8310=DIRECTION('ref_axis',(5.9211894646675E-15,7.40148683083438E-16,1.));
#8311=DIRECTION('center_axis',(-0.052263633556273,-0.0525535553916586,0.997249535684621));
#8312=DIRECTION('ref_axis',(-0.108857570442347,0.992963419871597,0.0466226999892949));
#8313=DIRECTION('center_axis',(0.,1.,0.));
#8314=DIRECTION('ref_axis',(0.998629534754574,0.,0.0523359562429438));
#8315=DIRECTION('center_axis',(0.375013085403515,-0.833398400816333,-0.405970801034895));
#8316=DIRECTION('ref_axis',(-0.565498005700927,-0.552672692935682,0.612180447279637));
#8317=DIRECTION('center_axis',(0.0522645732252408,0.0522112666801459,0.997267465636596));
#8318=DIRECTION('ref_axis',(-0.0228456520015352,-0.998308458201847,0.0534630570326489));
#8319=DIRECTION('center_axis',(-4.07418268117644E-12,-1.,-7.77400366303027E-11));
#8320=DIRECTION('ref_axis',(-0.998629534754574,0.,0.0523359562429438));
#8321=DIRECTION('center_axis',(-5.42947651131849E-20,1.,-1.03600583455278E-18));
#8322=DIRECTION('ref_axis',(-0.688354575693754,0.,0.725374371012288));
#8323=DIRECTION('center_axis',(-0.361627795167436,-0.818371417997736,-0.446647019431131));
#8324=DIRECTION('ref_axis',(0.514966362801185,-0.574689674697896,0.636035708886651));
#8325=DIRECTION('center_axis',(-0.0522636335562752,0.0525535553916633,0.99724953568462));
#8326=DIRECTION('ref_axis',(0.998629534754574,0.,0.0523359562429442));
#8327=DIRECTION('center_axis',(0.,-1.,0.));
#8328=DIRECTION('ref_axis',(0.,0.,1.));
#8329=DIRECTION('center_axis',(-5.42947651131849E-20,-1.,1.03600583455278E-18));
#8330=DIRECTION('ref_axis',(0.688354575693754,0.,0.725374371012288));
#8331=DIRECTION('',(5.42947651131849E-20,1.,-1.03600583455278E-18));
#8332=DIRECTION('center_axis',(-0.998629534754574,0.,-0.0523359562429438));
#8333=DIRECTION('ref_axis',(-0.0523359562429438,0.,0.998629534754574));
#8334=DIRECTION('center_axis',(-0.375013085256251,-0.833398400631247,0.405970801550885));
#8335=DIRECTION('ref_axis',(-0.565498005067695,0.552672693214781,0.612180447612612));
#8336=DIRECTION('center_axis',(-7.78474640228738E-11,1.,0.));
#8337=DIRECTION('ref_axis',(0.,0.,1.));
#8338=DIRECTION('center_axis',(-0.999738255790058,-0.0228783720979604,1.69987959829136E-9));
#8339=DIRECTION('ref_axis',(-0.022845652001536,0.998308458201847,0.0534630570326489));
#8340=DIRECTION('center_axis',(0.0522645732252412,-0.0522112666801462,0.997267465636596));
#8341=DIRECTION('ref_axis',(-0.998629534754574,0.,0.0523359562429445));
#8342=DIRECTION('center_axis',(0.361627795167442,-0.818371417997735,0.446647019431129));
#8343=DIRECTION('ref_axis',(0.514966362801186,0.574689674697898,0.636035708886649));
#8344=DIRECTION('center_axis',(0.994044372876412,0.108976074221546,-5.96658356591051E-15));
#8345=DIRECTION('ref_axis',(5.9211894646675E-15,7.40148683083438E-16,1.));
#8346=DIRECTION('center_axis',(0.,1.,0.));
#8347=DIRECTION('ref_axis',(0.998629534754574,0.,0.0523359562429438));
#8348=DIRECTION('center_axis',(-0.052263633556273,-0.0525535553916586,0.997249535684621));
#8349=DIRECTION('ref_axis',(-0.108857570442347,0.992963419871597,0.0466226999892949));
#8350=DIRECTION('center_axis',(0.375013085403515,-0.833398400816333,-0.405970801034895));
#8351=DIRECTION('ref_axis',(-0.565498005700926,-0.552672692935682,0.612180447279637));
#8352=DIRECTION('center_axis',(-0.999738255753194,0.0228783737088345,0.));
#8353=DIRECTION('ref_axis',(0.,0.,1.));
#8354=DIRECTION('center_axis',(-4.07418268117644E-12,-1.,-7.77400366303027E-11));
#8355=DIRECTION('ref_axis',(-0.998629534754574,0.,0.0523359562429438));
#8356=DIRECTION('center_axis',(0.0522645732252408,0.0522112666801459,0.997267465636596));
#8357=DIRECTION('ref_axis',(-0.0228456520015352,-0.998308458201847,0.0534630570326489));
#8358=DIRECTION('center_axis',(-5.42947651131849E-20,1.,-1.03600583455278E-18));
#8359=DIRECTION('ref_axis',(-0.688354575693754,0.,0.725374371012288));
#8360=DIRECTION('',(5.42947651131849E-20,-1.,1.03600583455278E-18));
#8361=DIRECTION('',(-5.42947651131849E-20,1.,-1.03600583455278E-18));
#8362=DIRECTION('center_axis',(-0.361627795167436,-0.818371417997736,-0.446647019431131));
#8363=DIRECTION('ref_axis',(0.51496636280118,-0.574689674697898,0.636035708886653));
#8364=DIRECTION('center_axis',(-0.0522636335562752,0.0525535553916633,0.99724953568462));
#8365=DIRECTION('ref_axis',(0.998629534754574,0.,0.0523359562429441));
#8366=DIRECTION('center_axis',(0.,-1.,0.));
#8367=DIRECTION('ref_axis',(0.,0.,1.));
#8368=DIRECTION('center_axis',(0.994044372876412,-0.108976074221552,-1.1933167131821E-14));
#8369=DIRECTION('ref_axis',(-0.108857570442347,-0.992963419871597,0.0466226999892957));
#8370=DIRECTION('center_axis',(-5.42947651131849E-20,-1.,1.03600583455278E-18));
#8371=DIRECTION('ref_axis',(0.688354575693754,0.,0.725374371012288));
#8372=DIRECTION('',(5.42947651131849E-20,1.,-1.03600583455278E-18));
#8373=DIRECTION('',(-5.42947651131849E-20,-1.,1.03600583455278E-18));
#8374=DIRECTION('center_axis',(0.998629534754574,0.,-0.0523359562429438));
#8375=DIRECTION('ref_axis',(-0.0523359562429438,0.,-0.998629534754574));
#8376=DIRECTION('center_axis',(-9.61618982193066E-33,1.03600583455278E-18,
1.));
#8377=DIRECTION('ref_axis',(1.,0.,9.61618982193066E-33));
#8378=DIRECTION('center_axis',(-0.998629534754574,0.,-0.0523359562429438));
#8379=DIRECTION('ref_axis',(-0.0523359562429438,0.,0.998629534754574));
#11241=CARTESIAN_POINT('',(0.,0.,0.));
#11242=CARTESIAN_POINT('Origin',(6.87409734069396,-2.22251806091942E-16,
0.7));
#11243=CARTESIAN_POINT('',(3.31825992066485,1.2493322588334,0.7));
#11244=CARTESIAN_POINT('',(4.3,1.27917501057225,0.7));
#11245=CARTESIAN_POINT('Ctrl Pts',(3.31826243508713,1.24933270901874,0.7));
#11246=CARTESIAN_POINT('Ctrl Pts',(3.64552542112514,1.25866821321074,0.7));
#11247=CARTESIAN_POINT('Ctrl Pts',(3.97277304530853,1.26856018917077,0.7));
#11248=CARTESIAN_POINT('Ctrl Pts',(4.30000000005992,1.27917501058303,0.7));
#11249=CARTESIAN_POINT('',(4.3,-1.27917501057184,0.7));
#11250=CARTESIAN_POINT('',(4.3,0.742407407407408,0.7));
#11251=CARTESIAN_POINT('',(3.31825992075695,-1.24933225883136,0.7));
#11252=CARTESIAN_POINT('Ctrl Pts',(4.3000000000599,-1.27917501058303,0.7));
#11253=CARTESIAN_POINT('Ctrl Pts',(3.97277304533917,-1.26856018917177,0.7));
#11254=CARTESIAN_POINT('Ctrl Pts',(3.64552542118644,-1.25866821321259,0.7));
#11255=CARTESIAN_POINT('Ctrl Pts',(3.3182624351791,-1.24933270902137,0.7));
#11256=CARTESIAN_POINT('',(3.26759951430388,-1.24789152572578,0.7));
#11257=CARTESIAN_POINT('Ctrl Pts',(3.26760216044043,-1.24789199949781,0.7));
#11258=CARTESIAN_POINT('Ctrl Pts',(3.27154046708102,-1.24840675231115,0.699999999449966));
#11259=CARTESIAN_POINT('Ctrl Pts',(3.27549053112987,-1.2488275353013,0.699997549264952));
#11260=CARTESIAN_POINT('Ctrl Pts',(3.27944900419773,-1.24915404112413,0.699995443099811));
#11261=CARTESIAN_POINT('Ctrl Pts',(3.28202272903949,-1.24936632907779,0.699994073710794));
#11262=CARTESIAN_POINT('Ctrl Pts',(3.28459959180148,-1.24953872742098,0.699992815093061));
#11263=CARTESIAN_POINT('Ctrl Pts',(3.28717866899733,-1.24967118132558,0.699992046536556));
#11264=CARTESIAN_POINT('Ctrl Pts',(3.28888409507617,-1.24975876704947,0.699991538325205));
#11265=CARTESIAN_POINT('Ctrl Pts',(3.29059037034979,-1.2498288805585,0.699991238158591));
#11266=CARTESIAN_POINT('Ctrl Pts',(3.29229723346923,-1.24988151179005,0.69999118215758));
#11267=CARTESIAN_POINT('Ctrl Pts',(3.29393274317941,-1.24993194283473,0.699991128497625));
#11268=CARTESIAN_POINT('Ctrl Pts',(3.29556870469678,-1.24996631998408,0.699991298652463));
#11269=CARTESIAN_POINT('Ctrl Pts',(3.29720488848534,-1.24998463806557,0.699991673963628));
#11270=CARTESIAN_POINT('Ctrl Pts',(3.29943508678369,-1.25000960650399,0.699992185531049));
#11271=CARTESIAN_POINT('Ctrl Pts',(3.30166551218918,-1.25000473681137,0.699993084765318));
#11272=CARTESIAN_POINT('Ctrl Pts',(3.30389557412726,-1.24997002667259,0.699994176731177));
#11273=CARTESIAN_POINT('Ctrl Pts',(3.30868977915254,-1.24989540653807,0.699996524248132));
#11274=CARTESIAN_POINT('Ctrl Pts',(3.31348068594496,-1.24968290539118,0.699999999312134));
#11275=CARTESIAN_POINT('Ctrl Pts',(3.3182624351791,-1.24933270902137,0.7));
#11276=CARTESIAN_POINT('',(1.1,-1.19266190204492,0.7));
#11277=CARTESIAN_POINT('Ctrl Pts',(3.26760216044045,-1.24789199949781,0.7));
#11278=CARTESIAN_POINT('Ctrl Pts',(2.54512260523322,-1.2274084473838,0.7));
#11279=CARTESIAN_POINT('Ctrl Pts',(1.82256951666701,-1.20959509718369,0.7));
#11280=CARTESIAN_POINT('Ctrl Pts',(1.09999999999999,-1.19266190204553,0.7));
#11281=CARTESIAN_POINT('',(1.1,1.19266190204492,0.7));
#11282=CARTESIAN_POINT('',(1.1,-0.696450594095222,0.7));
#11283=CARTESIAN_POINT('',(3.26759952419083,1.24789152650872,0.7));
#11284=CARTESIAN_POINT('Ctrl Pts',(1.09999999999999,1.19266190204553,0.7));
#11285=CARTESIAN_POINT('Ctrl Pts',(1.82256951996781,1.20959509726105,0.7));
#11286=CARTESIAN_POINT('Ctrl Pts',(2.54512261183467,1.22740844754655,0.7));
#11287=CARTESIAN_POINT('Ctrl Pts',(3.26760217034162,1.24789199977852,0.7));
#11288=CARTESIAN_POINT('Ctrl Pts',(3.3182624351791,1.24933270902137,0.7));
#11289=CARTESIAN_POINT('Ctrl Pts',(3.3143012451848,1.2496228108833,0.699999999430174));
#11290=CARTESIAN_POINT('Ctrl Pts',(3.31033365565543,1.24981842655856,0.699997549220164));
#11291=CARTESIAN_POINT('Ctrl Pts',(3.30636302717881,1.24991943948955,0.699995443052606));
#11292=CARTESIAN_POINT('Ctrl Pts',(3.30378139908369,1.24998511620097,0.699994073661998));
#11293=CARTESIAN_POINT('Ctrl Pts',(3.3011989045204,1.25001078941611,0.699992815050698));
#11294=CARTESIAN_POINT('Ctrl Pts',(3.29861646861803,1.2499964568765,0.699992046505716));
#11295=CARTESIAN_POINT('Ctrl Pts',(3.2969088217217,1.24998697942277,0.699991538302026));
#11296=CARTESIAN_POINT('Ctrl Pts',(3.29520131971864,1.24996000972381,0.699991238145114));
#11297=CARTESIAN_POINT('Ctrl Pts',(3.29349422410899,1.24991555258537,0.699991182154076));
#11298=CARTESIAN_POINT('Ctrl Pts',(3.29185849176351,1.24987295392896,0.699991128503682));
#11299=CARTESIAN_POINT('Ctrl Pts',(3.29022322047391,1.2498143016413,0.699991298668259));
#11300=CARTESIAN_POINT('Ctrl Pts',(3.28858863969825,1.2497396036024,0.699991673987721));
#11301=CARTESIAN_POINT('Ctrl Pts',(3.286360626573,1.24963778654105,0.699992185566407));
#11302=CARTESIAN_POINT('Ctrl Pts',(3.28413408201674,1.24950616665997,0.699993084809042));
#11303=CARTESIAN_POINT('Ctrl Pts',(3.2819095957713,1.24934477520901,0.699994176777649));
#11304=CARTESIAN_POINT('Ctrl Pts',(3.27712738077041,1.24899781481787,0.699996524298861));
#11305=CARTESIAN_POINT('Ctrl Pts',(3.27235629258357,1.24851338385513,0.699999999330822));
#11306=CARTESIAN_POINT('Ctrl Pts',(3.26760217026193,1.24789200078152,0.699999999999999));
#11307=CARTESIAN_POINT('',(3.15,1.,0.7));
#11308=CARTESIAN_POINT('Origin',(3.3,1.,0.7));
#11309=CARTESIAN_POINT('',(3.15,-1.,0.7));
#11310=CARTESIAN_POINT('Origin',(3.3,-1.,0.7));
#11311=CARTESIAN_POINT('',(1.6,-4.89858719658941E-17,0.7));
#11312=CARTESIAN_POINT('Origin',(2.,0.,0.7));
#11313=CARTESIAN_POINT('Origin',(9.9,-1.,0.8));
#11314=CARTESIAN_POINT('',(9.75,-1.,0.9));
#11315=CARTESIAN_POINT('Origin',(9.9,-1.,0.9));
#11316=CARTESIAN_POINT('',(9.75,-1.,0.7));
#11317=CARTESIAN_POINT('',(9.75,-1.,0.8));
#11318=CARTESIAN_POINT('Origin',(9.9,-1.,0.7));
#11319=CARTESIAN_POINT('Origin',(3.3,-1.,0.8));
#11320=CARTESIAN_POINT('',(3.15,-1.,0.9));
#11321=CARTESIAN_POINT('Origin',(3.3,-1.,0.9));
#11322=CARTESIAN_POINT('',(3.15,-1.,0.8));
#11323=CARTESIAN_POINT('Origin',(3.3,1.,0.8));
#11324=CARTESIAN_POINT('',(3.15,1.,0.9));
#11325=CARTESIAN_POINT('Origin',(3.3,1.,0.9));
#11326=CARTESIAN_POINT('',(3.15,1.,0.8));
#11327=CARTESIAN_POINT('Origin',(9.9,1.,0.8));
#11328=CARTESIAN_POINT('',(9.75,1.,0.9));
#11329=CARTESIAN_POINT('Origin',(9.9,1.,0.9));
#11330=CARTESIAN_POINT('',(9.75,1.,0.7));
#11331=CARTESIAN_POINT('',(9.75,1.,0.8));
#11332=CARTESIAN_POINT('Origin',(9.9,1.,0.7));
#11333=CARTESIAN_POINT('Origin',(11.3732050807569,0.3,0.9));
#11334=CARTESIAN_POINT('',(11.3732050807569,0.3,0.9));
#11335=CARTESIAN_POINT('',(11.5464101615138,0.,0.9));
#11336=CARTESIAN_POINT('',(10.8757685185329,1.16158539931442,0.9));
#11337=CARTESIAN_POINT('',(11.3732050807569,0.3,0.6));
#11338=CARTESIAN_POINT('',(11.3732050807569,0.3,0.9));
#11339=CARTESIAN_POINT('',(11.5464101615138,0.,0.6));
#11340=CARTESIAN_POINT('',(11.5464101615138,0.,0.6));
#11341=CARTESIAN_POINT('',(11.5464101615138,0.,0.9));
#11342=CARTESIAN_POINT('Origin',(11.0267949192431,0.3,0.9));
#11343=CARTESIAN_POINT('',(11.0267949192431,0.3,0.9));
#11344=CARTESIAN_POINT('',(8.95044612996854,0.3,0.9));
#11345=CARTESIAN_POINT('',(11.0267949192431,0.3,0.6));
#11346=CARTESIAN_POINT('',(11.0267949192431,0.3,0.9));
#11347=CARTESIAN_POINT('',(11.3732050807569,0.3,0.6));
#11348=CARTESIAN_POINT('Origin',(10.8535898384862,5.55111512312578E-17,
0.9));
#11349=CARTESIAN_POINT('',(10.8535898384862,4.24230095489963E-17,0.9));
#11350=CARTESIAN_POINT('',(10.3561532762622,-0.86158539931442,0.9));
#11351=CARTESIAN_POINT('',(10.8535898384862,5.55111512312578E-17,0.6));
#11352=CARTESIAN_POINT('',(10.8535898384862,4.24230095489963E-17,0.9));
#11353=CARTESIAN_POINT('',(11.0267949192431,0.3,0.6));
#11354=CARTESIAN_POINT('Origin',(11.0267949192431,-0.3,0.9));
#11355=CARTESIAN_POINT('',(11.0267949192431,-0.3,0.9));
#11356=CARTESIAN_POINT('',(10.4427558166406,0.71158539931442,0.9));
#11357=CARTESIAN_POINT('',(11.0267949192431,-0.3,0.6));
#11358=CARTESIAN_POINT('',(11.0267949192431,-0.3,0.9));
#11359=CARTESIAN_POINT('',(10.8535898384862,4.24230095489963E-17,0.6));
#11360=CARTESIAN_POINT('Origin',(11.3732050807569,-0.3,0.9));
#11361=CARTESIAN_POINT('',(11.3732050807569,-0.3,0.9));
#11362=CARTESIAN_POINT('',(9.12365121072543,-0.3,0.9));
#11363=CARTESIAN_POINT('',(11.3732050807569,-0.3,0.6));
#11364=CARTESIAN_POINT('',(11.3732050807569,-0.3,0.9));
#11365=CARTESIAN_POINT('',(11.0267949192431,-0.3,0.6));
#11366=CARTESIAN_POINT('Origin',(11.5464101615138,0.,0.9));
#11367=CARTESIAN_POINT('',(10.9623710589113,-1.01158539931442,0.9));
#11368=CARTESIAN_POINT('',(11.3732050807569,-0.3,0.6));
#11369=CARTESIAN_POINT('Origin',(11.2,5.55111512312578E-17,0.6));
#11370=CARTESIAN_POINT('',(11.03,-2.0818995585505E-17,0.6));
#11371=CARTESIAN_POINT('Origin',(11.2,0.,0.6));
#11372=CARTESIAN_POINT('Origin',(2.17320508075689,0.3,0.9));
#11373=CARTESIAN_POINT('',(2.17320508075689,0.3,0.9));
#11374=CARTESIAN_POINT('',(2.34641016151378,0.,0.9));
#11375=CARTESIAN_POINT('',(2.82576851853285,-0.830273029389787,0.9));
#11376=CARTESIAN_POINT('',(2.17320508075689,0.3,0.6));
#11377=CARTESIAN_POINT('',(2.17320508075689,0.3,0.9));
#11378=CARTESIAN_POINT('',(2.34641016151378,0.,0.6));
#11379=CARTESIAN_POINT('',(2.34641016151378,0.,0.6));
#11380=CARTESIAN_POINT('',(2.34641016151378,0.,0.9));
#11381=CARTESIAN_POINT('Origin',(1.82679491924311,0.3,0.9));
#11382=CARTESIAN_POINT('',(1.82679491924311,0.3,0.9));
#11383=CARTESIAN_POINT('',(4.35044612996854,0.3,0.9));
#11384=CARTESIAN_POINT('',(1.82679491924311,0.3,0.6));
#11385=CARTESIAN_POINT('',(1.82679491924311,0.3,0.9));
#11386=CARTESIAN_POINT('',(2.17320508075689,0.3,0.6));
#11387=CARTESIAN_POINT('Origin',(1.65358983848622,5.55111512312578E-17,
0.9));
#11388=CARTESIAN_POINT('',(1.65358983848622,4.24230095489963E-17,0.9));
#11389=CARTESIAN_POINT('',(2.30615327626219,1.13027302938979,0.9));
#11390=CARTESIAN_POINT('',(1.65358983848622,5.55111512312578E-17,0.6));
#11391=CARTESIAN_POINT('',(1.65358983848622,4.24230095489963E-17,0.9));
#11392=CARTESIAN_POINT('',(1.82679491924311,0.3,0.6));
#11393=CARTESIAN_POINT('Origin',(1.82679491924311,-0.3,0.9));
#11394=CARTESIAN_POINT('',(1.82679491924311,-0.3,0.9));
#11395=CARTESIAN_POINT('',(2.39275581664063,-1.28027302938979,0.9));
#11396=CARTESIAN_POINT('',(1.82679491924311,-0.3,0.6));
#11397=CARTESIAN_POINT('',(1.82679491924311,-0.3,0.9));
#11398=CARTESIAN_POINT('',(1.65358983848622,4.24230095489963E-17,0.6));
#11399=CARTESIAN_POINT('Origin',(2.17320508075689,-0.3,0.9));
#11400=CARTESIAN_POINT('',(2.17320508075689,-0.3,0.9));
#11401=CARTESIAN_POINT('',(4.52365121072543,-0.3,0.9));
#11402=CARTESIAN_POINT('',(2.17320508075689,-0.3,0.6));
#11403=CARTESIAN_POINT('',(2.17320508075689,-0.3,0.9));
#11404=CARTESIAN_POINT('',(1.82679491924311,-0.3,0.6));
#11405=CARTESIAN_POINT('Origin',(2.34641016151378,0.,0.9));
#11406=CARTESIAN_POINT('',(2.9123710589113,0.980273029389787,0.9));
#11407=CARTESIAN_POINT('',(2.17320508075689,-0.3,0.6));
#11408=CARTESIAN_POINT('Origin',(2.,5.55111512312578E-17,0.6));
#11409=CARTESIAN_POINT('',(1.83,-2.0818995585505E-17,0.6));
#11410=CARTESIAN_POINT('Origin',(2.,0.,0.6));
#11411=CARTESIAN_POINT('Origin',(2.,0.,0.45));
#11412=CARTESIAN_POINT('',(1.83,-2.0818995585505E-17,0.32));
#11413=CARTESIAN_POINT('',(1.83,2.0818995585505E-17,0.45));
#11414=CARTESIAN_POINT('Origin',(2.,0.,0.32));
#11415=CARTESIAN_POINT('Origin',(11.2,0.,0.45));
#11416=CARTESIAN_POINT('',(11.03,-2.0818995585505E-17,0.32));
#11417=CARTESIAN_POINT('',(11.03,2.0818995585505E-17,0.45));
#11418=CARTESIAN_POINT('Origin',(11.2,0.,0.32));
#11419=CARTESIAN_POINT('Origin',(12.4,-0.72,0.32));
#11420=CARTESIAN_POINT('',(0.200274469199584,-0.72,0.));
#11421=CARTESIAN_POINT('',(0.217044958570157,-0.72,0.32));
#11422=CARTESIAN_POINT('',(0.225070308370679,-0.72,0.473132796510599));
#11423=CARTESIAN_POINT('',(0.,-0.72,0.));
#11424=CARTESIAN_POINT('',(9.63649764092939,-0.72,0.));
#11425=CARTESIAN_POINT('',(0.0167704893705732,-0.72,0.32));
#11426=CARTESIAN_POINT('',(0.0253444014197637,-0.72,0.483599987759188));
#11427=CARTESIAN_POINT('',(-0.1,-0.72,0.32));
#11428=CARTESIAN_POINT('Origin',(12.4,-0.72,0.32));
#11429=CARTESIAN_POINT('',(0.9,-0.72,0.32));
#11430=CARTESIAN_POINT('',(0.9,-0.72,0.));
#11431=CARTESIAN_POINT('',(0.9,-0.72,0.16));
#11432=CARTESIAN_POINT('',(1.1,-0.72,0.32));
#11433=CARTESIAN_POINT('',(-0.1,-0.72,0.32));
#11434=CARTESIAN_POINT('',(1.1,-0.72,0.));
#11435=CARTESIAN_POINT('',(1.1,-0.72,0.16));
#11436=CARTESIAN_POINT('',(9.63649764092939,-0.72,0.));
#11437=CARTESIAN_POINT('Origin',(12.4,-0.72,0.32));
#11438=CARTESIAN_POINT('',(4.3,-0.72,0.32));
#11439=CARTESIAN_POINT('',(4.3,-0.72,0.));
#11440=CARTESIAN_POINT('',(4.3,-0.72,0.16));
#11441=CARTESIAN_POINT('',(4.5,-0.72,0.32));
#11442=CARTESIAN_POINT('',(-0.1,-0.72,0.32));
#11443=CARTESIAN_POINT('',(4.5,-0.72,0.));
#11444=CARTESIAN_POINT('',(4.5,-0.72,0.16));
#11445=CARTESIAN_POINT('',(9.63649764092939,-0.72,0.));
#11446=CARTESIAN_POINT('Origin',(12.4,-0.72,0.32));
#11447=CARTESIAN_POINT('',(8.7,-0.72,0.32));
#11448=CARTESIAN_POINT('',(8.7,-0.72,0.));
#11449=CARTESIAN_POINT('',(8.7,-0.72,0.16));
#11450=CARTESIAN_POINT('',(8.9,-0.72,0.32));
#11451=CARTESIAN_POINT('',(-0.1,-0.72,0.32));
#11452=CARTESIAN_POINT('',(8.9,-0.72,0.));
#11453=CARTESIAN_POINT('',(8.9,-0.72,0.16));
#11454=CARTESIAN_POINT('',(9.63649764092939,-0.72,0.));
#11455=CARTESIAN_POINT('Origin',(-0.0999999999999996,0.72,0.32));
#11456=CARTESIAN_POINT('',(0.217044958570158,0.72,0.32));
#11457=CARTESIAN_POINT('',(0.200274469199584,0.72,0.));
#11458=CARTESIAN_POINT('',(0.207951231396534,0.72,0.146481348799182));
#11459=CARTESIAN_POINT('',(0.0167704893705736,0.72,0.32));
#11460=CARTESIAN_POINT('',(12.4,0.72,0.32));
#11461=CARTESIAN_POINT('',(0.,0.72,0.));
#11462=CARTESIAN_POINT('',(0.00822532444561912,0.72,0.156948540047771));
#11463=CARTESIAN_POINT('',(3.38649764092939,0.72,0.));
#11464=CARTESIAN_POINT('Origin',(-0.0999999999999996,0.72,0.32));
#11465=CARTESIAN_POINT('',(0.9,0.72,0.));
#11466=CARTESIAN_POINT('',(0.9,0.72,0.32));
#11467=CARTESIAN_POINT('',(0.9,0.72,0.16));
#11468=CARTESIAN_POINT('',(1.1,0.72,0.));
#11469=CARTESIAN_POINT('',(3.38649764092939,0.72,0.));
#11470=CARTESIAN_POINT('',(1.1,0.72,0.32));
#11471=CARTESIAN_POINT('',(1.1,0.72,0.16));
#11472=CARTESIAN_POINT('',(12.4,0.72,0.32));
#11473=CARTESIAN_POINT('Origin',(-0.0999999999999996,0.72,0.32));
#11474=CARTESIAN_POINT('',(4.3,0.72,0.));
#11475=CARTESIAN_POINT('',(4.3,0.72,0.32));
#11476=CARTESIAN_POINT('',(4.3,0.72,0.16));
#11477=CARTESIAN_POINT('',(4.5,0.72,0.));
#11478=CARTESIAN_POINT('',(3.38649764092939,0.72,0.));
#11479=CARTESIAN_POINT('',(4.5,0.72,0.32));
#11480=CARTESIAN_POINT('',(4.5,0.72,0.16));
#11481=CARTESIAN_POINT('',(12.4,0.72,0.32));
#11482=CARTESIAN_POINT('Origin',(6.15,0.,0.32));
#11483=CARTESIAN_POINT('',(1.6,-4.89858719658941E-17,0.32));
#11484=CARTESIAN_POINT('Origin',(2.,0.,0.32));
#11485=CARTESIAN_POINT('Origin',(6.15,0.,0.32));
#11486=CARTESIAN_POINT('',(10.8,-4.89858719658942E-17,0.32));
#11487=CARTESIAN_POINT('Origin',(11.2,0.,0.32));
#11488=CARTESIAN_POINT('Origin',(6.15,0.,0.32));
#11489=CARTESIAN_POINT('',(0.217044958570157,-0.75,0.32));
#11490=CARTESIAN_POINT('',(0.0167704893705736,-0.75,0.32));
#11491=CARTESIAN_POINT('Origin',(6.15,0.,0.32));
#11492=CARTESIAN_POINT('',(0.9,0.696450594095222,0.32));
#11493=CARTESIAN_POINT('',(1.1,-0.696450594095222,0.32));
#11494=CARTESIAN_POINT('Origin',(6.15,0.,0.32));
#11495=CARTESIAN_POINT('',(4.3,0.742407407407408,0.32));
#11496=CARTESIAN_POINT('',(4.5,-0.742407407407408,0.32));
#11497=CARTESIAN_POINT('Origin',(6.15,0.,0.32));
#11498=CARTESIAN_POINT('',(8.7,0.72,0.32));
#11499=CARTESIAN_POINT('',(8.7,0.844259259259259,0.32));
#11500=CARTESIAN_POINT('',(8.9,0.72,0.32));
#11501=CARTESIAN_POINT('',(12.4,0.72,0.32));
#11502=CARTESIAN_POINT('',(8.9,-0.844259259259259,0.32));
#11503=CARTESIAN_POINT('Origin',(-0.0999999999999996,0.72,0.32));
#11504=CARTESIAN_POINT('',(8.7,0.72,0.));
#11505=CARTESIAN_POINT('',(8.7,0.72,0.16));
#11506=CARTESIAN_POINT('',(8.9,0.72,0.));
#11507=CARTESIAN_POINT('',(3.38649764092939,0.72,0.));
#11508=CARTESIAN_POINT('',(8.9,0.72,0.16));
#11509=CARTESIAN_POINT('Origin',(12.4,1.99376954809806,0.));
#11510=CARTESIAN_POINT('',(12.4,1.91212902562343,0.));
#11511=CARTESIAN_POINT('',(12.4,-1.91212902562343,0.));
#11512=CARTESIAN_POINT('',(12.4,1.99376954809806,0.));
#11513=CARTESIAN_POINT('',(12.4,-1.8833055216247,0.604732563714112));
#11514=CARTESIAN_POINT('Ctrl Pts',(12.4,-1.8833055216247,0.604732563714112));
#11515=CARTESIAN_POINT('Ctrl Pts',(12.4,-1.88809880980762,0.504101072758768));
#11516=CARTESIAN_POINT('Ctrl Pts',(12.4,-1.89289370245628,0.403468941627095));
#11517=CARTESIAN_POINT('Ctrl Pts',(12.4,-1.90250151416087,0.201891903194028));
#11518=CARTESIAN_POINT('Ctrl Pts',(12.4,-1.90731451170285,0.100945553925438));
#11519=CARTESIAN_POINT('Ctrl Pts',(12.4,-1.91212902562343,0.));
#11520=CARTESIAN_POINT('',(12.4,-1.78288409287054,0.7));
#11521=CARTESIAN_POINT('Ctrl Pts',(12.4000000030461,-1.78288409409899,0.7));
#11522=CARTESIAN_POINT('Ctrl Pts',(12.4000000066823,-1.79082830277209,0.699999997040196));
#11523=CARTESIAN_POINT('Ctrl Pts',(12.4000021328137,-1.79871128857748,0.699006690321208));
#11524=CARTESIAN_POINT('Ctrl Pts',(12.4000039827682,-1.8063921320806,0.697119229445379));
#11525=CARTESIAN_POINT('Ctrl Pts',(12.4000049365067,-1.81035196808589,0.69614615460905));
#11526=CARTESIAN_POINT('Ctrl Pts',(12.4000058167808,-1.81425808325963,0.694934510320783));
#11527=CARTESIAN_POINT('Ctrl Pts',(12.400006432968,-1.81808986884151,0.693492707237305));
#11528=CARTESIAN_POINT('Ctrl Pts',(12.4000076352846,-1.82556652433459,0.690679432664999));
#11529=CARTESIAN_POINT('Ctrl Pts',(12.4000076271954,-1.83268048852469,0.687023315130674));
#11530=CARTESIAN_POINT('Ctrl Pts',(12.4000063864816,-1.83928589538344,0.682605693351404));
#11531=CARTESIAN_POINT('Ctrl Pts',(12.4000055969106,-1.84348947395919,0.679794387301037));
#11532=CARTESIAN_POINT('Ctrl Pts',(12.400004329084,-1.84748689691167,0.676673627174617));
#11533=CARTESIAN_POINT('Ctrl Pts',(12.4000032503406,-1.8512341074341,0.673255429390325));
#11534=CARTESIAN_POINT('Ctrl Pts',(12.4000023796213,-1.85425870830395,0.670496394655072));
#11535=CARTESIAN_POINT('Ctrl Pts',(12.4000016297172,-1.85710218072175,0.667559826261508));
#11536=CARTESIAN_POINT('Ctrl Pts',(12.4000016274617,-1.859744520612,0.664455546516084));
#11537=CARTESIAN_POINT('Ctrl Pts',(12.4000016230979,-1.86485672743849,0.658449612092435));
#11538=CARTESIAN_POINT('Ctrl Pts',(12.4000041080363,-1.86921906069885,0.651817317967817));
#11539=CARTESIAN_POINT('Ctrl Pts',(12.40000495371,-1.8727702927896,0.64472299566344));
#11540=CARTESIAN_POINT('Ctrl Pts',(12.4000050555652,-1.8731980125259,0.643868536819953));
#11541=CARTESIAN_POINT('Ctrl Pts',(12.4000051394069,-1.87361391018412,0.643007349425002));
#11542=CARTESIAN_POINT('Ctrl Pts',(12.4000052029357,-1.87401783114888,0.642139703315781));
#11543=CARTESIAN_POINT('Ctrl Pts',(12.4000057294153,-1.87736522853405,0.634949295858174));
#11544=CARTESIAN_POINT('Ctrl Pts',(12.4000043880804,-1.87985460663586,0.627401584261416));
#11545=CARTESIAN_POINT('Ctrl Pts',(12.4000025112034,-1.88143175301701,0.619663949188762));
#11546=CARTESIAN_POINT('Ctrl Pts',(12.4000013193515,-1.88243327046239,0.614750406220363));
#11547=CARTESIAN_POINT('Ctrl Pts',(12.4,-1.88306607129604,0.609759643802656));
#11548=CARTESIAN_POINT('Ctrl Pts',(12.4,-1.8833055216247,0.604732563714112));
#11549=CARTESIAN_POINT('',(12.4,1.78288409287164,0.7));
#11550=CARTESIAN_POINT('',(12.4,0.99688477404903,0.7));
#11551=CARTESIAN_POINT('',(12.4,1.8833055216247,0.604732563714112));
#11552=CARTESIAN_POINT('Ctrl Pts',(12.4,1.8833055216247,0.604732563714112));
#11553=CARTESIAN_POINT('Ctrl Pts',(12.4,1.88292893537322,0.612638709665068));
#11554=CARTESIAN_POINT('Ctrl Pts',(12.4000029905988,1.88158186833012,0.620459457162159));
#11555=CARTESIAN_POINT('Ctrl Pts',(12.400004351969,1.87934739482834,0.62803467841275));
#11556=CARTESIAN_POINT('Ctrl Pts',(12.4000050124983,1.87826324073514,0.631710133556493));
#11557=CARTESIAN_POINT('Ctrl Pts',(12.4000053733669,1.87696936339782,0.63532777623417));
#11558=CARTESIAN_POINT('Ctrl Pts',(12.4000053391329,1.87547104796815,0.638868146717817));
#11559=CARTESIAN_POINT('Ctrl Pts',(12.4000052683671,1.872373843052,0.646186534188034));
#11560=CARTESIAN_POINT('Ctrl Pts',(12.4000032465668,1.86844110215533,0.653093304890266));
#11561=CARTESIAN_POINT('Ctrl Pts',(12.4000021327941,1.86374151467895,0.659427433016556));
#11562=CARTESIAN_POINT('Ctrl Pts',(12.4000018304335,1.86246569800928,0.66114698527342));
#11563=CARTESIAN_POINT('Ctrl Pts',(12.4000016226794,1.86113309763036,0.662824214875179));
#11564=CARTESIAN_POINT('Ctrl Pts',(12.400001625255,1.85974452038344,0.664455546516227));
#11565=CARTESIAN_POINT('Ctrl Pts',(12.4000016287814,1.85784336180007,0.666689070188443));
#11566=CARTESIAN_POINT('Ctrl Pts',(12.400002024929,1.85583728779192,0.668836587948716));
#11567=CARTESIAN_POINT('Ctrl Pts',(12.4000025639666,1.85373364862045,0.670894373083513));
#11568=CARTESIAN_POINT('Ctrl Pts',(12.400004021536,1.84804536272624,0.676458668669153));
#11569=CARTESIAN_POINT('Ctrl Pts',(12.4000062945443,1.84171268252251,0.681305055194542));
#11570=CARTESIAN_POINT('Ctrl Pts',(12.4000070319583,1.83490078417639,0.685381489016216));
#11571=CARTESIAN_POINT('Ctrl Pts',(12.4000075068619,1.8305138392177,0.688006761722114));
#11572=CARTESIAN_POINT('Ctrl Pts',(12.4000074483741,1.82592714021755,0.69031203082117));
#11573=CARTESIAN_POINT('Ctrl Pts',(12.4000068708525,1.82117863971551,0.692273867243687));
#11574=CARTESIAN_POINT('Ctrl Pts',(12.4000059767178,1.81382688138917,0.695311236040001));
#11575=CARTESIAN_POINT('Ctrl Pts',(12.4000038254996,1.80617119073902,0.697493343451155));
#11576=CARTESIAN_POINT('Ctrl Pts',(12.4000020685374,1.7983596509798,0.698751345219246));
#11577=CARTESIAN_POINT('Ctrl Pts',(12.4000009204513,1.79325520389048,0.699573385900268));
#11578=CARTESIAN_POINT('Ctrl Pts',(12.400000005426,1.78808359082883,0.699999998062804));
#11579=CARTESIAN_POINT('Ctrl Pts',(12.4000000030461,1.78288409409899,0.7));
#11580=CARTESIAN_POINT('Ctrl Pts',(12.4,1.91212902562343,0.));
#11581=CARTESIAN_POINT('Ctrl Pts',(12.4,1.90731404243129,0.1009553931071));
#11582=CARTESIAN_POINT('Ctrl Pts',(12.4,1.9025005759122,0.201911581737034));
#11583=CARTESIAN_POINT('Ctrl Pts',(12.4,1.89289276481806,0.403488620176902));
#11584=CARTESIAN_POINT('Ctrl Pts',(12.4,1.88809834114759,0.504110911924693));
#11585=CARTESIAN_POINT('Ctrl Pts',(12.4,1.8833055216247,0.604732563714112));
#11586=CARTESIAN_POINT('Origin',(8.9,-1.68851851851852,0.));
#11587=CARTESIAN_POINT('',(8.9,1.62420669932031,0.));
#11588=CARTESIAN_POINT('',(8.9,-1.68851851851852,0.));
#11589=CARTESIAN_POINT('',(8.9,1.59320117118329,0.605106081470792));
#11590=CARTESIAN_POINT('Ctrl Pts',(8.9,1.59320117118329,0.605106081470792));
#11591=CARTESIAN_POINT('Ctrl Pts',(8.9,1.59837103562161,0.504197738990529));
#11592=CARTESIAN_POINT('Ctrl Pts',(8.9,1.60354126123154,0.403288838380538));
#11593=CARTESIAN_POINT('Ctrl Pts',(8.9,1.61387642009944,0.201587196710533));
#11594=CARTESIAN_POINT('Ctrl Pts',(8.9,1.61904141157348,0.100793304842659));
#11595=CARTESIAN_POINT('Ctrl Pts',(8.9,1.62420669932031,0.));
#11596=CARTESIAN_POINT('',(8.9,1.49312521822106,0.7));
#11597=CARTESIAN_POINT('Ctrl Pts',(8.9,1.49312521822106,0.7));
#11598=CARTESIAN_POINT('Ctrl Pts',(8.9,1.50104136823484,0.7));
#11599=CARTESIAN_POINT('Ctrl Pts',(8.90000131173634,1.50889623314995,0.699007530025307));
#11600=CARTESIAN_POINT('Ctrl Pts',(8.90000245364087,1.51654949575132,0.697121675771258));
#11601=CARTESIAN_POINT('Ctrl Pts',(8.9000030153269,1.52031402289636,0.696194051841344));
#11602=CARTESIAN_POINT('Ctrl Pts',(8.90000353645954,1.52402976767023,0.695049421358208));
#11603=CARTESIAN_POINT('Ctrl Pts',(8.90000391188735,1.52767894577544,0.693695149285802));
#11604=CARTESIAN_POINT('Ctrl Pts',(8.90000468147812,1.53515940869299,0.690919022244083));
#11605=CARTESIAN_POINT('Ctrl Pts',(8.90000470661952,1.54227958804117,0.687295426711095));
#11606=CARTESIAN_POINT('Ctrl Pts',(8.9000039635008,1.54889410374269,0.682907715777054));
#11607=CARTESIAN_POINT('Ctrl Pts',(8.90000349228854,1.55308837416723,0.680125464281631));
#11608=CARTESIAN_POINT('Ctrl Pts',(8.90000272405863,1.55707914411963,0.677034908766328));
#11609=CARTESIAN_POINT('Ctrl Pts',(8.90000205379677,1.56082314136721,0.673648333128258));
#11610=CARTESIAN_POINT('Ctrl Pts',(8.90000149471997,1.56394607304962,0.670823532879853));
#11611=CARTESIAN_POINT('Ctrl Pts',(8.90000100172653,1.56687805273397,0.667809941545923));
#11612=CARTESIAN_POINT('Ctrl Pts',(8.90000100003,1.56959740049228,0.664618488856983));
#11613=CARTESIAN_POINT('Ctrl Pts',(8.90000099684156,1.57470809805256,0.658620525035968));
#11614=CARTESIAN_POINT('Ctrl Pts',(8.90000253934467,1.57907071782202,0.651995745956818));
#11615=CARTESIAN_POINT('Ctrl Pts',(8.90000305932469,1.58262507990443,0.644909256877938));
#11616=CARTESIAN_POINT('Ctrl Pts',(8.90000311559331,1.58300970826793,0.644142406277414));
#11617=CARTESIAN_POINT('Ctrl Pts',(8.9000031627798,1.58338482682255,0.643370127200485));
#11618=CARTESIAN_POINT('Ctrl Pts',(8.90000319981124,1.58375032531468,0.642592615892991));
#11619=CARTESIAN_POINT('Ctrl Pts',(8.90000354178946,1.58712563340961,0.635412448897651));
#11620=CARTESIAN_POINT('Ctrl Pts',(8.90000272882427,1.58964525157545,0.627871187463612));
#11621=CARTESIAN_POINT('Ctrl Pts',(8.90000156924769,1.59125549206429,0.620136848214628));
#11622=CARTESIAN_POINT('Ctrl Pts',(8.90000082792478,1.59228492658837,0.615192247765769));
#11623=CARTESIAN_POINT('Ctrl Pts',(8.89999999997262,1.59294182914154,0.610168076493048));
#11624=CARTESIAN_POINT('Ctrl Pts',(8.9000000009702,1.5932011715731,0.605106081469384));
#11625=CARTESIAN_POINT('',(8.9,-1.49312521822001,0.7));
#11626=CARTESIAN_POINT('',(8.9,-0.844259259259259,0.7));
#11627=CARTESIAN_POINT('',(8.9,-1.59320117118329,0.605106081470792));
#11628=CARTESIAN_POINT('Ctrl Pts',(8.90000000097019,-1.5932011715731,0.605106081469384));
#11629=CARTESIAN_POINT('Ctrl Pts',(8.89999999941083,-1.59279578158415,0.613018716877257));
#11630=CARTESIAN_POINT('Ctrl Pts',(8.90000185372291,-1.59142151714118,0.620841302874248));
#11631=CARTESIAN_POINT('Ctrl Pts',(8.90000269095591,-1.58916270068609,0.628413601005994));
#11632=CARTESIAN_POINT('Ctrl Pts',(8.90000316003867,-1.58789713677684,0.632656188846207));
#11633=CARTESIAN_POINT('Ctrl Pts',(8.90000337414869,-1.58635289833986,0.636820251299613));
#11634=CARTESIAN_POINT('Ctrl Pts',(8.90000326408749,-1.58453800492682,0.640875626603871));
#11635=CARTESIAN_POINT('Ctrl Pts',(8.9000030675631,-1.58129734600662,0.648116871770122));
#11636=CARTESIAN_POINT('Ctrl Pts',(8.90000169351568,-1.5772322800227,0.654932667693845));
#11637=CARTESIAN_POINT('Ctrl Pts',(8.90000116172667,-1.57240747726376,0.66116027211862));
#11638=CARTESIAN_POINT('Ctrl Pts',(8.90000106146602,-1.57149783490479,0.662334391157823));
#11639=CARTESIAN_POINT('Ctrl Pts',(8.90000099955281,-1.57056105641498,0.663487533005214));
#11640=CARTESIAN_POINT('Ctrl Pts',(8.90000100072893,-1.56959740053727,0.664618488856962));
#11641=CARTESIAN_POINT('Ctrl Pts',(8.9000010030487,-1.56769671285427,0.666849154291726));
#11642=CARTESIAN_POINT('Ctrl Pts',(8.90000124864079,-1.56569149899762,0.668993559652069));
#11643=CARTESIAN_POINT('Ctrl Pts',(8.90000158179872,-1.56358911460694,0.671047966011734));
#11644=CARTESIAN_POINT('Ctrl Pts',(8.90000248280001,-1.55790336961918,0.676603957919834));
#11645=CARTESIAN_POINT('Ctrl Pts',(8.90000387848177,-1.55157399841983,0.681441805123218));
#11646=CARTESIAN_POINT('Ctrl Pts',(8.90000432886686,-1.54476515293017,0.68550782533293));
#11647=CARTESIAN_POINT('Ctrl Pts',(8.9000046162921,-1.54041990676133,0.688102664467623));
#11648=CARTESIAN_POINT('Ctrl Pts',(8.90000458123012,-1.53587841548674,0.69038248607508));
#11649=CARTESIAN_POINT('Ctrl Pts',(8.90000422571091,-1.53117752164703,0.692323975790708));
#11650=CARTESIAN_POINT('Ctrl Pts',(8.90000367147839,-1.52384911813356,0.695350638493274));
#11651=CARTESIAN_POINT('Ctrl Pts',(8.9000023358238,-1.51621796414731,0.697522741667433));
#11652=CARTESIAN_POINT('Ctrl Pts',(8.90000125519218,-1.50843132129101,0.698770821080692));
#11653=CARTESIAN_POINT('Ctrl Pts',(8.90000055451733,-1.5033825102871,0.699580068042664));
#11654=CARTESIAN_POINT('Ctrl Pts',(8.9,-1.49826772866746,0.7));
#11655=CARTESIAN_POINT('Ctrl Pts',(8.9,-1.49312521822106,0.7));
#11656=CARTESIAN_POINT('',(8.9,-1.62420669932031,0.));
#11657=CARTESIAN_POINT('Ctrl Pts',(8.9,-1.62420669932031,0.));
#11658=CARTESIAN_POINT('Ctrl Pts',(8.9,-1.61904139377919,0.100793652073202));
#11659=CARTESIAN_POINT('Ctrl Pts',(8.9,-1.61387638451174,0.201587891198165));
#11660=CARTESIAN_POINT('Ctrl Pts',(8.9,-1.60354122564866,0.403289532862703));
#11661=CARTESIAN_POINT('Ctrl Pts',(8.9,-1.59837101783099,0.50419808623799));
#11662=CARTESIAN_POINT('Ctrl Pts',(8.9,-1.59320117118329,0.605106081470792));
#11663=CARTESIAN_POINT('',(8.9,-1.68851851851852,0.));
#11664=CARTESIAN_POINT('Origin',(4.5,-1.48481481481482,0.));
#11665=CARTESIAN_POINT('',(4.5,1.41772989878425,0.));
#11666=CARTESIAN_POINT('',(4.5,-1.48481481481482,0.));
#11667=CARTESIAN_POINT('',(4.5,1.38566996325095,0.605286533624017));
#11668=CARTESIAN_POINT('Ctrl Pts',(4.5,1.38566996325095,0.605286533624017));
#11669=CARTESIAN_POINT('Ctrl Pts',(4.5,1.3910232158183,0.504222354021684));
#11670=CARTESIAN_POINT('Ctrl Pts',(4.5,1.39637635187357,0.403158168247774));
#11671=CARTESIAN_POINT('Ctrl Pts',(4.5,1.4070629957395,0.201395990303158));
#11672=CARTESIAN_POINT('Ctrl Pts',(4.5,1.41239650438775,0.100697998177668));
#11673=CARTESIAN_POINT('Ctrl Pts',(4.5,1.41772989878425,0.));
#11674=CARTESIAN_POINT('',(4.5,1.28575421950843,0.7));
#11675=CARTESIAN_POINT('Ctrl Pts',(4.5,1.28575421950843,0.7));
#11676=CARTESIAN_POINT('Ctrl Pts',(4.5,1.29366545802379,0.7));
#11677=CARTESIAN_POINT('Ctrl Pts',(4.50000067540813,1.30151306508378,0.699006020085879));
#11678=CARTESIAN_POINT('Ctrl Pts',(4.50000126278178,1.30915682219698,0.697118891599074));
#11679=CARTESIAN_POINT('Ctrl Pts',(4.50000159346398,1.31346013814185,0.696056467716811));
#11680=CARTESIAN_POINT('Ctrl Pts',(4.50000189442328,1.31769890045703,0.694709922559592));
#11681=CARTESIAN_POINT('Ctrl Pts',(4.50000208642664,1.32184639782974,0.693090275295953));
#11682=CARTESIAN_POINT('Ctrl Pts',(4.50000243009859,1.32927011415192,0.690191225399894));
#11683=CARTESIAN_POINT('Ctrl Pts',(4.50000235826664,1.33632110693134,0.686451804482762));
#11684=CARTESIAN_POINT('Ctrl Pts',(4.50000192249634,1.34285330390028,0.681953677325188));
#11685=CARTESIAN_POINT('Ctrl Pts',(4.5000016824508,1.3464515866709,0.679475868782656));
#11686=CARTESIAN_POINT('Ctrl Pts',(4.50000134086274,1.34989218134371,0.676766953538005));
#11687=CARTESIAN_POINT('Ctrl Pts',(4.50000103767597,1.35314674504257,0.67383503027087));
#11688=CARTESIAN_POINT('Ctrl Pts',(4.50000074242034,1.35631617169348,0.670979804009792));
#11689=CARTESIAN_POINT('Ctrl Pts',(4.50000047986374,1.35928994516467,0.667930335702103));
#11690=CARTESIAN_POINT('Ctrl Pts',(4.5000004798165,1.36204555935344,0.66469809744354));
#11691=CARTESIAN_POINT('Ctrl Pts',(4.5000004797289,1.36715559606013,0.658704204607119));
#11692=CARTESIAN_POINT('Ctrl Pts',(4.50000128456446,1.3715183542993,0.652083197653858));
#11693=CARTESIAN_POINT('Ctrl Pts',(4.50000155892095,1.37507421485048,0.645000595057188));
#11694=CARTESIAN_POINT('Ctrl Pts',(4.50000158702893,1.37543851484667,0.644274978272754));
#11695=CARTESIAN_POINT('Ctrl Pts',(4.50000161091379,1.37579430519483,0.643544496675346));
#11696=CARTESIAN_POINT('Ctrl Pts',(4.50000163009343,1.37614149316233,0.642809317076966));
#11697=CARTESIAN_POINT('Ctrl Pts',(4.50000181728783,1.37953006709248,0.635633923185928));
#11698=CARTESIAN_POINT('Ctrl Pts',(4.50000140772507,1.38206400387968,0.628095594687559));
#11699=CARTESIAN_POINT('Ctrl Pts',(4.50000081194859,1.38368993781387,0.620362729373495));
#11700=CARTESIAN_POINT('Ctrl Pts',(4.50000042990035,1.38473258588096,0.615403944208116));
#11701=CARTESIAN_POINT('Ctrl Pts',(4.49999999988018,1.38540098970406,0.610364492806037));
#11702=CARTESIAN_POINT('Ctrl Pts',(4.50000000014037,1.38566996330298,0.605286533623957));
#11703=CARTESIAN_POINT('',(4.5,-1.28575421950842,0.7));
#11704=CARTESIAN_POINT('',(4.5,-0.742407407407408,0.7));
#11705=CARTESIAN_POINT('',(4.5,-1.38566996325095,0.605286533624017));
#11706=CARTESIAN_POINT('Ctrl Pts',(4.50000000014037,-1.38566996330298,0.605286533623957));
#11707=CARTESIAN_POINT('Ctrl Pts',(4.49999999973491,-1.38525081272033,0.613199687771457));
#11708=CARTESIAN_POINT('Ctrl Pts',(4.50000095642016,-1.38386419754969,0.62102180968747));
#11709=CARTESIAN_POINT('Ctrl Pts',(4.50000138305812,-1.38159414679432,0.628592503408469));
#11710=CARTESIAN_POINT('Ctrl Pts',(4.50000162118259,-1.38032713666619,0.632818023740444));
#11711=CARTESIAN_POINT('Ctrl Pts',(4.50000172745986,-1.37878391728058,0.636965253716347));
#11712=CARTESIAN_POINT('Ctrl Pts',(4.50000166716583,-1.37697237493585,0.641004309729874));
#11713=CARTESIAN_POINT('Ctrl Pts',(4.50000155916287,-1.37372741146613,0.648239354085419));
#11714=CARTESIAN_POINT('Ctrl Pts',(4.50000084040372,-1.36965973349804,0.655049237033139));
#11715=CARTESIAN_POINT('Ctrl Pts',(4.50000056390271,-1.36483316768901,0.661270759279915));
#11716=CARTESIAN_POINT('Ctrl Pts',(4.50000051219424,-1.36393055121024,0.662434246679675));
#11717=CARTESIAN_POINT('Ctrl Pts',(4.50000048023544,-1.3630012658104,0.663577087492372));
#11718=CARTESIAN_POINT('Ctrl Pts',(4.50000048056391,-1.36204555937839,0.664698097443534));
#11719=CARTESIAN_POINT('Ctrl Pts',(4.50000048121673,-1.36014610273268,0.666926093123284));
#11720=CARTESIAN_POINT('Ctrl Pts',(4.50000060829837,-1.35814231322364,0.669067903674665));
#11721=CARTESIAN_POINT('Ctrl Pts',(4.50000078085101,-1.35604151212276,0.671119765431539));
#11722=CARTESIAN_POINT('Ctrl Pts',(4.50000124774248,-1.3503571825734,0.676671675324794));
#11723=CARTESIAN_POINT('Ctrl Pts',(4.50000197143062,-1.34402953514766,0.681505303070731));
#11724=CARTESIAN_POINT('Ctrl Pts',(4.50000220836427,-1.33722229030693,0.685566265232058));
#11725=CARTESIAN_POINT('Ctrl Pts',(4.50000235894787,-1.33289593407788,0.688147216755564));
#11726=CARTESIAN_POINT('Ctrl Pts',(4.50000234488938,-1.32837489877041,0.690415387400166));
#11727=CARTESIAN_POINT('Ctrl Pts',(4.50000216490635,-1.32369554581057,0.69234752884452));
#11728=CARTESIAN_POINT('Ctrl Pts',(4.50000188343739,-1.31637767466938,0.695369135087455));
#11729=CARTESIAN_POINT('Ctrl Pts',(4.50000119588393,-1.3087575932273,0.697536490026807));
#11730=CARTESIAN_POINT('Ctrl Pts',(4.50000064127173,-1.30098224657147,0.698779892333419));
#11731=CARTESIAN_POINT('Ctrl Pts',(4.50000028296845,-1.29595903898196,0.699583183579437));
#11732=CARTESIAN_POINT('Ctrl Pts',(4.5,-1.29087043558603,0.7));
#11733=CARTESIAN_POINT('Ctrl Pts',(4.5,-1.28575421950843,0.7));
#11734=CARTESIAN_POINT('',(4.5,-1.41772989878425,0.));
#11735=CARTESIAN_POINT('Ctrl Pts',(4.5,-1.41772989878425,0.));
#11736=CARTESIAN_POINT('Ctrl Pts',(4.5,-1.41239649634988,0.100698149937961));
#11737=CARTESIAN_POINT('Ctrl Pts',(4.5,-1.40706297966336,0.201396293824709));
#11738=CARTESIAN_POINT('Ctrl Pts',(4.5,-1.39637633579674,0.403158471769294));
#11739=CARTESIAN_POINT('Ctrl Pts',(4.5,-1.39102320777973,0.504222505781934));
#11740=CARTESIAN_POINT('Ctrl Pts',(4.5,-1.38566996325095,0.605286533624017));
#11741=CARTESIAN_POINT('',(4.5,-1.48481481481482,0.));
#11742=CARTESIAN_POINT('Origin',(1.1,-1.39290118819044,0.));
#11743=CARTESIAN_POINT('',(1.1,1.324891758307,0.));
#11744=CARTESIAN_POINT('',(1.1,-1.39290118819044,0.));
#11745=CARTESIAN_POINT('',(1.10000000295569,1.29254692766489,0.605334652628491));
#11746=CARTESIAN_POINT('Ctrl Pts',(1.10000000295569,1.29254692766489,0.605334652628491));
#11747=CARTESIAN_POINT('Ctrl Pts',(1.10000000295569,1.29794978210809,0.504228164786351));
#11748=CARTESIAN_POINT('Ctrl Pts',(1.1,1.30335245345465,0.403121008362245));
#11749=CARTESIAN_POINT('Ctrl Pts',(1.1,1.31413403739463,0.20134322693425));
#11750=CARTESIAN_POINT('Ctrl Pts',(1.1,1.31951302132877,0.100671299071668));
#11751=CARTESIAN_POINT('Ctrl Pts',(1.1,1.324891758307,0.));
#11752=CARTESIAN_POINT('Ctrl Pts',(1.1,1.19266190204553,0.7));
#11753=CARTESIAN_POINT('Ctrl Pts',(1.1,1.20057109129252,0.7));
#11754=CARTESIAN_POINT('Ctrl Pts',(1.10000046829629,1.20841685974333,0.699006220526237));
#11755=CARTESIAN_POINT('Ctrl Pts',(1.10000087277688,1.21605887983377,0.697119382842322));
#11756=CARTESIAN_POINT('Ctrl Pts',(1.10000109992184,1.22035042410288,0.696059787689036));
#11757=CARTESIAN_POINT('Ctrl Pts',(1.10000130563842,1.22457776983048,0.694717521940989));
#11758=CARTESIAN_POINT('Ctrl Pts',(1.10000143498593,1.22871439246446,0.693103507978966));
#11759=CARTESIAN_POINT('Ctrl Pts',(1.10000166711622,1.23613807995602,0.690206957744321));
#11760=CARTESIAN_POINT('Ctrl Pts',(1.10000160692769,1.24318920265812,0.686469797174223));
#11761=CARTESIAN_POINT('Ctrl Pts',(1.10000129432656,1.24972159507123,0.681973692132557));
#11762=CARTESIAN_POINT('Ctrl Pts',(1.10000112259081,1.25331033895651,0.679503636989594));
#11763=CARTESIAN_POINT('Ctrl Pts',(1.10000088087184,1.25674225826706,0.676803638555143));
#11764=CARTESIAN_POINT('Ctrl Pts',(1.10000066684112,1.25998923415267,0.673881729486736));
#11765=CARTESIAN_POINT('Ctrl Pts',(1.100000457217,1.26316935916797,0.671019978599686));
#11766=CARTESIAN_POINT('Ctrl Pts',(1.1000002715704,1.26615273734033,0.667962699881477));
#11767=CARTESIAN_POINT('Ctrl Pts',(1.1000002731257,1.2689166530284,0.664721467295484));
#11768=CARTESIAN_POINT('Ctrl Pts',(1.10000027600127,1.2740268283512,0.658728785663437));
#11769=CARTESIAN_POINT('Ctrl Pts',(1.10000085014601,1.27838972527875,0.652108677049879));
#11770=CARTESIAN_POINT('Ctrl Pts',(1.1000010530947,1.28194599975408,0.64502688444408));
#11771=CARTESIAN_POINT('Ctrl Pts',(1.10000107362034,1.2823056710724,0.644310652415237));
#11772=CARTESIAN_POINT('Ctrl Pts',(1.10000109127028,1.28265705236355,0.643589678557342));
#11773=CARTESIAN_POINT('Ctrl Pts',(1.10000110571348,1.28300005475086,0.642864123553892));
#11774=CARTESIAN_POINT('Ctrl Pts',(1.10000124853573,1.28639184812822,0.635689442715943));
#11775=CARTESIAN_POINT('Ctrl Pts',(1.10000097361067,1.28892914698194,0.628151301589031));
#11776=CARTESIAN_POINT('Ctrl Pts',(1.10000056283738,1.29055881622654,0.620418355899457));
#11777=CARTESIAN_POINT('Ctrl Pts',(1.10000029930222,1.29160434466024,0.615457217544876));
#11778=CARTESIAN_POINT('Ctrl Pts',(1.0999999999818,1.29227543558766,0.610415225971447));
#11779=CARTESIAN_POINT('Ctrl Pts',(1.1000000000255,1.29254692753179,0.605334652628598));
#11780=CARTESIAN_POINT('',(1.10000000295569,-1.29254692766489,0.605334652628491));
#11781=CARTESIAN_POINT('Ctrl Pts',(1.1000000000255,-1.29254692753179,0.605334652628598));
#11782=CARTESIAN_POINT('Ctrl Pts',(1.09999999995744,-1.29212405100831,0.613248166229861));
#11783=CARTESIAN_POINT('Ctrl Pts',(1.10000066442022,-1.29073420569755,0.621070584654331));
#11784=CARTESIAN_POINT('Ctrl Pts',(1.10000095378343,-1.28846118610397,0.628641296001913));
#11785=CARTESIAN_POINT('Ctrl Pts',(1.10000111506646,-1.28719426797524,0.632861000698125));
#11786=CARTESIAN_POINT('Ctrl Pts',(1.10000118318417,-1.28565198202118,0.637002542581089));
#11787=CARTESIAN_POINT('Ctrl Pts',(1.10000113489265,-1.28384214455607,0.641036116698538));
#11788=CARTESIAN_POINT('Ctrl Pts',(1.10000104828677,-1.28059638744501,0.648269916488365));
#11789=CARTESIAN_POINT('Ctrl Pts',(1.10000053334783,-1.27652829029495,0.655078571385522));
#11790=CARTESIAN_POINT('Ctrl Pts',(1.10000033433257,-1.27170133822839,0.661298646557671));
#11791=CARTESIAN_POINT('Ctrl Pts',(1.10000029715544,-1.27079963749419,0.662460590217389));
#11792=CARTESIAN_POINT('Ctrl Pts',(1.10000027400485,-1.26987132743055,0.663601924550879));
#11793=CARTESIAN_POINT('Ctrl Pts',(1.10000027368829,-1.26891665304159,0.664721467295481));
#11794=CARTESIAN_POINT('Ctrl Pts',(1.10000027305905,-1.2670190620795,0.666946764442229));
#11795=CARTESIAN_POINT('Ctrl Pts',(1.10000036187052,-1.26501734165944,0.669086014589825));
#11796=CARTESIAN_POINT('Ctrl Pts',(1.10000048327469,-1.26291879257262,0.671135465892351));
#11797=CARTESIAN_POINT('Ctrl Pts',(1.10000081209565,-1.25723491092676,0.676686367091516));
#11798=CARTESIAN_POINT('Ctrl Pts',(1.10000132622062,-1.25090760500066,0.68151881845922));
#11799=CARTESIAN_POINT('Ctrl Pts',(1.10000150097561,-1.24410063152763,0.68557843671136));
#11800=CARTESIAN_POINT('Ctrl Pts',(1.10000161196703,-1.2397773464179,0.688156805381407));
#11801=CARTESIAN_POINT('Ctrl Pts',(1.1000016084534,-1.23525961544019,0.690422742497405));
#11802=CARTESIAN_POINT('Ctrl Pts',(1.10000148831111,-1.23058375131837,0.692353039195786));
#11803=CARTESIAN_POINT('Ctrl Pts',(1.10000130031927,-1.22326722442338,0.695373457954986));
#11804=CARTESIAN_POINT('Ctrl Pts',(1.1000008264887,-1.21564857658641,0.697539632783775));
#11805=CARTESIAN_POINT('Ctrl Pts',(1.10000044322439,-1.20787483729518,0.698781928831272));
#11806=CARTESIAN_POINT('Ctrl Pts',(1.1000001958084,-1.20285650563037,0.6995838921283));
#11807=CARTESIAN_POINT('Ctrl Pts',(1.1,-1.19777295102175,0.7));
#11808=CARTESIAN_POINT('Ctrl Pts',(1.1,-1.19266190204553,0.7));
#11809=CARTESIAN_POINT('',(1.1,-1.324891758307,0.));
#11810=CARTESIAN_POINT('Ctrl Pts',(1.1,-1.324891758307,0.));
#11811=CARTESIAN_POINT('Ctrl Pts',(1.1,-1.3195129727271,0.10067220872632));
#11812=CARTESIAN_POINT('Ctrl Pts',(1.1,-1.31413394019217,0.201345046154956));
#11813=CARTESIAN_POINT('Ctrl Pts',(1.1,-1.30335235623932,0.40312282767794));
#11814=CARTESIAN_POINT('Ctrl Pts',(1.10000000295569,-1.29794973349953,0.504229074424201));
#11815=CARTESIAN_POINT('Ctrl Pts',(1.10000000295569,-1.29254692766489,0.605334652628491));
#11816=CARTESIAN_POINT('',(1.1,-1.39290118819044,0.));
#11817=CARTESIAN_POINT('Origin',(0.199725906950915,-1.5,-0.0104671912485888));
#11818=CARTESIAN_POINT('',(0.200274469199584,1.20659878095028,0.));
#11819=CARTESIAN_POINT('',(0.200274469199585,-0.75,0.));
#11820=CARTESIAN_POINT('',(0.231993417893744,1.17491202960101,0.605233595624295));
#11821=CARTESIAN_POINT('Ctrl Pts',(0.200274469199584,1.20659878095028,-9.43255890062389E-18));
#11822=CARTESIAN_POINT('Ctrl Pts',(0.210847451958254,1.19603647956141,0.20174452921517));
#11823=CARTESIAN_POINT('Ctrl Pts',(0.221420434855641,1.18547422886796,0.403489061077219));
#11824=CARTESIAN_POINT('Ctrl Pts',(0.231993417893744,1.17491202960101,0.605233595624295));
#11825=CARTESIAN_POINT('',(0.231993417893744,-1.17491202960101,0.605233595624295));
#11826=CARTESIAN_POINT('',(0.231993417893744,-0.75,0.605233595624295));
#11827=CARTESIAN_POINT('',(0.200274469199584,-1.20659878095028,1.38777878078145E-17));
#11828=CARTESIAN_POINT('Ctrl Pts',(0.231993417893744,-1.17491202960101,
0.605233595624295));
#11829=CARTESIAN_POINT('Ctrl Pts',(0.221420434855641,-1.18547422886796,
0.40348906107722));
#11830=CARTESIAN_POINT('Ctrl Pts',(0.210847451958254,-1.19603647956141,
0.20174452921517));
#11831=CARTESIAN_POINT('Ctrl Pts',(0.200274469199584,-1.20659878095028,
2.0491421059976E-17));
#11832=CARTESIAN_POINT('',(0.200274469199585,-0.75,0.));
#11833=CARTESIAN_POINT('Origin',(6.87299528185878,-3.57834294608796E-18,
0.));
#11834=CARTESIAN_POINT('Ctrl Pts',(8.90000000000001,-1.62420669932031,-3.75133951679985E-17));
#11835=CARTESIAN_POINT('Ctrl Pts',(10.0682843079684,-1.69891080436391,-1.31961514553165E-7));
#11836=CARTESIAN_POINT('Ctrl Pts',(11.2345361392062,-1.79243531443695,-6.44452192334729E-8));
#11837=CARTESIAN_POINT('Ctrl Pts',(12.4000000002382,-1.91212902541327,2.95121624705651E-11));
#11838=CARTESIAN_POINT('Ctrl Pts',(12.4000000002382,1.91212902541327,2.95118849063386E-11));
#11839=CARTESIAN_POINT('Ctrl Pts',(11.2345361911441,1.79243531977099,-6.4445136166539E-8));
#11840=CARTESIAN_POINT('Ctrl Pts',(10.0682843567552,1.69891080748336,-1.31958638870612E-7));
#11841=CARTESIAN_POINT('Ctrl Pts',(8.9,1.62420669932031,6.39679281766448E-17));
#11842=CARTESIAN_POINT('',(8.7,1.61160179736194,0.));
#11843=CARTESIAN_POINT('',(8.7,1.68851851851852,0.));
#11844=CARTESIAN_POINT('Ctrl Pts',(8.70000000002062,1.61160179731554,-3.21507306454832E-13));
#11845=CARTESIAN_POINT('Ctrl Pts',(7.99734938728961,1.56795839277283,5.29471456843263E-9));
#11846=CARTESIAN_POINT('Ctrl Pts',(7.29393815910572,1.53097060499506,-6.44604909847991E-9));
#11847=CARTESIAN_POINT('Ctrl Pts',(6.58949465297818,1.49904250536939,-7.60372244394637E-9));
#11848=CARTESIAN_POINT('Ctrl Pts',(5.94302350041144,1.46974193664425,-8.66612477447903E-9));
#11849=CARTESIAN_POINT('Ctrl Pts',(5.29757001768168,1.44478244743454,1.79883147367388E-8));
#11850=CARTESIAN_POINT('Ctrl Pts',(4.65216233480351,1.42284617839366,3.84107779578714E-9));
#11851=CARTESIAN_POINT('Ctrl Pts',(4.60144142975536,1.4211222642714,2.72928337404163E-9));
#11852=CARTESIAN_POINT('Ctrl Pts',(4.55072080855761,1.41941704699729,1.44770501019496E-9));
#11853=CARTESIAN_POINT('Ctrl Pts',(4.50000000001737,1.41772989873549,-1.00876616052154E-12));
#11854=CARTESIAN_POINT('',(4.3,1.41116952203211,0.));
#11855=CARTESIAN_POINT('',(4.3,1.48481481481482,0.));
#11856=CARTESIAN_POINT('Ctrl Pts',(4.3,1.41116952203211,-1.0790522121662E-15));
#11857=CARTESIAN_POINT('Ctrl Pts',(3.23514221724601,1.37672428690534,3.20725535317031E-8));
#11858=CARTESIAN_POINT('Ctrl Pts',(2.16992716239601,1.34987955958158,4.63097810372671E-9));
#11859=CARTESIAN_POINT('Ctrl Pts',(1.10000000020726,1.32489175811528,-9.82792569252214E-12));
#11860=CARTESIAN_POINT('',(0.9,1.32024227787037,0.));
#11861=CARTESIAN_POINT('',(0.9,1.39290118819044,0.));
#11862=CARTESIAN_POINT('',(0.297857995688647,1.306435779838,0.));
#11863=CARTESIAN_POINT('Ctrl Pts',(0.9,1.32024227787037,-6.93889390390723E-18));
#11864=CARTESIAN_POINT('Ctrl Pts',(0.699470323836888,1.31560060380002,-4.72996299588896E-10));
#11865=CARTESIAN_POINT('Ctrl Pts',(0.498765843889866,1.3110112408976,-1.02277582142263E-13));
#11866=CARTESIAN_POINT('Ctrl Pts',(0.297857995688647,1.306435779838,-1.00157829096748E-16));
#11867=CARTESIAN_POINT('Ctrl Pts',(0.297857995688647,1.306435779838,-1.95156391047391E-17));
#11868=CARTESIAN_POINT('Ctrl Pts',(0.289922476296638,1.30625505685688,-1.46278605970555E-13));
#11869=CARTESIAN_POINT('Ctrl Pts',(0.282050301799808,1.30510306275878,-1.25203502999379E-6));
#11870=CARTESIAN_POINT('Ctrl Pts',(0.274405144964298,1.30305953674341,-1.39678564665046E-6));
#11871=CARTESIAN_POINT('Ctrl Pts',(0.269498922713003,1.30174811919849,-1.48967827287246E-6));
#11872=CARTESIAN_POINT('Ctrl Pts',(0.26468600784495,1.30006837070384,-1.17796618578504E-6));
#11873=CARTESIAN_POINT('Ctrl Pts',(0.260012701218123,1.29803054880949,-5.63923085528507E-7));
#11874=CARTESIAN_POINT('Ctrl Pts',(0.252740988282594,1.29485967708789,3.91534262267771E-7));
#11875=CARTESIAN_POINT('Ctrl Pts',(0.245891302634708,1.2908611961912,2.26944434681222E-6));
#11876=CARTESIAN_POINT('Ctrl Pts',(0.239629152465829,1.28609427281,1.73040332626933E-6));
#11877=CARTESIAN_POINT('Ctrl Pts',(0.238677421334952,1.28536978852616,1.6484790500646E-6));
#11878=CARTESIAN_POINT('Ctrl Pts',(0.23773930716971,1.28462746803483,1.50379952206709E-6));
#11879=CARTESIAN_POINT('Ctrl Pts',(0.236815449960777,1.28386742955246,1.27686598471174E-6));
#11880=CARTESIAN_POINT('Ctrl Pts',(0.233849259515119,1.28142720517261,5.48259784756267E-7));
#11881=CARTESIAN_POINT('Ctrl Pts',(0.231029859162728,1.27880446664625,-1.01231737317126E-6));
#11882=CARTESIAN_POINT('Ctrl Pts',(0.228365947504865,1.27601569667724,-2.73789903475208E-6));
#11883=CARTESIAN_POINT('Ctrl Pts',(0.222875659368053,1.2702680771449,-6.2943009513513E-6));
#11884=CARTESIAN_POINT('Ctrl Pts',(0.218108003769119,1.26388547870891,-1.02458913084139E-5));
#11885=CARTESIAN_POINT('Ctrl Pts',(0.214119068651703,1.25703104885628,-1.16727273233865E-5));
#11886=CARTESIAN_POINT('Ctrl Pts',(0.211608035823831,1.25271618840614,-1.25709199407453E-5));
#11887=CARTESIAN_POINT('Ctrl Pts',(0.209406266788438,1.24821342134138,-1.25531979180244E-5));
#11888=CARTESIAN_POINT('Ctrl Pts',(0.207536767894457,1.24355803714115,-1.16467700682383E-5));
#11889=CARTESIAN_POINT('Ctrl Pts',(0.204585779527196,1.23620955211972,-1.02159812889057E-5));
#11890=CARTESIAN_POINT('Ctrl Pts',(0.20249437279756,1.22856635796309,-6.44823334219156E-6));
#11891=CARTESIAN_POINT('Ctrl Pts',(0.201333199355162,1.22077498745768,-3.37414558979738E-6));
#11892=CARTESIAN_POINT('Ctrl Pts',(0.200635497716839,1.21609347152911,-1.5270519663277E-6));
#11893=CARTESIAN_POINT('Ctrl Pts',(0.200274469246579,1.21135795995708,-3.76748562593766E-12));
#11894=CARTESIAN_POINT('Ctrl Pts',(0.200274469199584,1.20659878095028,6.07153216591882E-18));
#11895=CARTESIAN_POINT('',(-2.81723893694256E-19,1.20714678905882,-2.77862675945125E-17));
#11896=CARTESIAN_POINT('',(0.,-1.5,0.));
#11897=CARTESIAN_POINT('',(0.292751161823634,1.50665779898694,0.));
#11898=CARTESIAN_POINT('Ctrl Pts',(0.292751161823634,1.50665779898694,-4.77048955893622E-17));
#11899=CARTESIAN_POINT('Ctrl Pts',(0.274916014309114,1.50625165707847,3.84528327419955E-12));
#11900=CARTESIAN_POINT('Ctrl Pts',(0.257184594685611,1.50420857033458,-2.03607170333744E-6));
#11901=CARTESIAN_POINT('Ctrl Pts',(0.239764500086274,1.50063675387888,-2.79213621391921E-6));
#11902=CARTESIAN_POINT('Ctrl Pts',(0.222116086584643,1.49701812291205,-3.55811018958082E-6));
#11903=CARTESIAN_POINT('Ctrl Pts',(0.204785660682177,1.49183000356027,-2.9511242418033E-6));
#11904=CARTESIAN_POINT('Ctrl Pts',(0.187998620502071,1.4851341555102,-6.80337370794577E-7));
#11905=CARTESIAN_POINT('Ctrl Pts',(0.185044527596802,1.48395585623842,-2.80736529130144E-7));
#11906=CARTESIAN_POINT('Ctrl Pts',(0.182107319868513,1.48273075079643,1.61255976403501E-7));
#11907=CARTESIAN_POINT('Ctrl Pts',(0.17918831289364,1.48145903083089,6.35063889779883E-7));
#11908=CARTESIAN_POINT('Ctrl Pts',(0.162608037952008,1.47423552404966,3.32634402063389E-6));
#11909=CARTESIAN_POINT('Ctrl Pts',(0.146760254055949,1.46557586252388,7.36741945499403E-6));
#11910=CARTESIAN_POINT('Ctrl Pts',(0.131860714325404,1.4555643673366,8.80872142158042E-6));
#11911=CARTESIAN_POINT('Ctrl Pts',(0.12416804976458,1.45039541073654,9.55286874158632E-6));
#11912=CARTESIAN_POINT('Ctrl Pts',(0.116728404005452,1.44486529627202,9.54902993357918E-6));
#11913=CARTESIAN_POINT('Ctrl Pts',(0.109574210210226,1.43898090192647,7.86258910610491E-6));
#11914=CARTESIAN_POINT('Ctrl Pts',(0.100675189791982,1.43166137062374,5.76484451217541E-6));
#11915=CARTESIAN_POINT('Ctrl Pts',(0.0922175942578585,1.42379373777092,
1.07962821494929E-6));
#11916=CARTESIAN_POINT('Ctrl Pts',(0.0842272493232774,1.41542759110015,
-4.17082519724513E-6));
#11917=CARTESIAN_POINT('Ctrl Pts',(0.0719003514327883,1.40252093480537,
-1.22708263387205E-5));
#11918=CARTESIAN_POINT('Ctrl Pts',(0.0607923942774574,1.38854365509349,
-2.1446290640466E-5));
#11919=CARTESIAN_POINT('Ctrl Pts',(0.0509667079859164,1.37370740939602,
-2.73088451608079E-5));
#11920=CARTESIAN_POINT('Ctrl Pts',(0.040988527714452,1.35864090617899,-3.32623861267576E-5));
#11921=CARTESIAN_POINT('Ctrl Pts',(0.0323319291028794,1.34268723517955,
-3.58272570146011E-5));
#11922=CARTESIAN_POINT('Ctrl Pts',(0.0251054147216294,1.32603775378173,
-3.42048160832586E-5));
#11923=CARTESIAN_POINT('Ctrl Pts',(0.0239557673766072,1.32338903116455,
-3.39467061825833E-5));
#11924=CARTESIAN_POINT('Ctrl Pts',(0.022842414085455,1.32072266145131,-3.35898145907185E-5));
#11925=CARTESIAN_POINT('Ctrl Pts',(0.0217659098422027,1.31803938112476,
-3.31388957009043E-5));
#11926=CARTESIAN_POINT('Ctrl Pts',(0.0146851456525434,1.30038996137917,
-3.01729526055095E-5));
#11927=CARTESIAN_POINT('Ctrl Pts',(0.00925910545076598,1.282173175788,-2.28911926108039E-5));
#11928=CARTESIAN_POINT('Ctrl Pts',(0.0055880418397064,1.26361786690427,
-1.53360241296986E-5));
#11929=CARTESIAN_POINT('Ctrl Pts',(0.00217213684284492,1.24635225152695,
-8.30598038733772E-6));
#11930=CARTESIAN_POINT('Ctrl Pts',(0.000275638047107462,1.2287919996398,
-1.11502351997496E-6));
#11931=CARTESIAN_POINT('Ctrl Pts',(2.78020181985954E-5,1.21111091902543,
-1.13803743790751E-7));
#11932=CARTESIAN_POINT('Ctrl Pts',(9.289355304618E-6,1.20979019141994,-3.90154078055202E-8));
#11933=CARTESIAN_POINT('Ctrl Pts',(3.5054796412911E-11,1.20846879032832,
-2.82152417201308E-12));
#11934=CARTESIAN_POINT('Ctrl Pts',(6.5594231435373E-18,1.20714678905882,
2.42861286636753E-17));
#11935=CARTESIAN_POINT('',(12.8678148030684,2.16300527278356,0.));
#11936=CARTESIAN_POINT('Ctrl Pts',(0.292751161823634,1.50665779898694,0.));
#11937=CARTESIAN_POINT('Ctrl Pts',(4.48443904223854,1.60211086545473,0.));
#11938=CARTESIAN_POINT('Ctrl Pts',(8.67612692265345,1.70561506876628,0.));
#11939=CARTESIAN_POINT('Ctrl Pts',(12.8678148030684,2.16300527278356,0.));
#11940=CARTESIAN_POINT('',(13.2,1.86519007666192,1.29914761427265E-16));
#11941=CARTESIAN_POINT('Ctrl Pts',(13.2,1.86519007666192,1.40512601554121E-16));
#11942=CARTESIAN_POINT('Ctrl Pts',(13.2000000013352,1.88296731840607,9.35191444695304E-11));
#11943=CARTESIAN_POINT('Ctrl Pts',(13.1983511006715,1.90064589040826,-4.81925060583158E-6));
#11944=CARTESIAN_POINT('Ctrl Pts',(13.1951709302004,1.91804121845656,-9.22684518112407E-6));
#11945=CARTESIAN_POINT('Ctrl Pts',(13.1919252271695,1.93579500539423,-1.37252653764835E-5));
#11946=CARTESIAN_POINT('Ctrl Pts',(13.1870840836913,1.95325521073227,-1.77396479500911E-5));
#11947=CARTESIAN_POINT('Ctrl Pts',(13.1807207319279,1.9702167899609,-1.88895599539727E-5));
#11948=CARTESIAN_POINT('Ctrl Pts',(13.179605107926,1.97319049715201,-1.90911627380646E-5));
#11949=CARTESIAN_POINT('Ctrl Pts',(13.1784425783122,1.97614882406338,-1.92137058190342E-5));
#11950=CARTESIAN_POINT('Ctrl Pts',(13.1772333926356,1.97909058504493,-1.92562174744009E-5));
#11951=CARTESIAN_POINT('Ctrl Pts',(13.1703491364924,1.99583891121373,-1.94982490583826E-5));
#11952=CARTESIAN_POINT('Ctrl Pts',(13.1620175712498,2.0119031422279,-1.67925698753361E-5));
#11953=CARTESIAN_POINT('Ctrl Pts',(13.1523342210936,2.02708796667103,-1.30402710852334E-5));
#11954=CARTESIAN_POINT('Ctrl Pts',(13.1443502942575,2.03960786168842,-9.94649893779315E-6));
#11955=CARTESIAN_POINT('Ctrl Pts',(13.1354462980072,2.05153020544825,-6.18593217696112E-6));
#11956=CARTESIAN_POINT('Ctrl Pts',(13.1256528604983,2.06273196126272,-4.73977425690188E-6));
#11957=CARTESIAN_POINT('Ctrl Pts',(13.1217453950533,2.06720132901318,-4.16277439392992E-6));
#11958=CARTESIAN_POINT('Ctrl Pts',(13.1176961215346,2.07155579183536,-3.97575052791371E-6));
#11959=CARTESIAN_POINT('Ctrl Pts',(13.1135113749213,2.07579033931164,-3.99023031318383E-6));
#11960=CARTESIAN_POINT('Ctrl Pts',(13.1009362730034,2.08851509208914,-4.03374185458576E-6));
#11961=CARTESIAN_POINT('Ctrl Pts',(13.0872516297578,2.10004749226926,-5.60236028337187E-6));
#11962=CARTESIAN_POINT('Ctrl Pts',(13.0726646436523,2.11028882659185,-6.03124820804926E-6));
#11963=CARTESIAN_POINT('Ctrl Pts',(13.0580194031224,2.12057106059247,-6.46184893473862E-6));
#11964=CARTESIAN_POINT('Ctrl Pts',(13.0424632957183,2.12955278528135,-5.76500392338198E-6));
#11965=CARTESIAN_POINT('Ctrl Pts',(13.0261754841647,2.13709349482706,-4.98347139369932E-6));
#11966=CARTESIAN_POINT('Ctrl Pts',(13.0233759049672,2.13838960594114,-4.84914013593099E-6));
#11967=CARTESIAN_POINT('Ctrl Pts',(13.0205546633935,2.13964302898522,-4.72077764982159E-6));
#11968=CARTESIAN_POINT('Ctrl Pts',(13.0177126224567,2.14085289970554,-4.61407510358037E-6));
#11969=CARTESIAN_POINT('Ctrl Pts',(13.0148367726024,2.14207716304734,-4.50610322390289E-6));
#11970=CARTESIAN_POINT('Ctrl Pts',(13.0119432782921,2.14325527660784,-4.42172619954107E-6));
#11971=CARTESIAN_POINT('Ctrl Pts',(13.0090331608036,2.14438664763146,-4.38057543634576E-6));
#11972=CARTESIAN_POINT('Ctrl Pts',(12.9922536897216,2.1509100294015,-4.14330390220891E-6));
#11973=CARTESIAN_POINT('Ctrl Pts',(12.9749229882599,2.15588345271621,-5.05640020348117E-6));
#11974=CARTESIAN_POINT('Ctrl Pts',(12.9572550825995,2.15928949382789,-4.85686529648217E-6));
#11975=CARTESIAN_POINT('Ctrl Pts',(12.9529252316797,2.16012420794307,-4.80796553341985E-6));
#11976=CARTESIAN_POINT('Ctrl Pts',(12.9485750628159,2.16086455090717,-4.70814629363608E-6));
#11977=CARTESIAN_POINT('Ctrl Pts',(12.944207640703,2.16150979950679,-4.55317442353944E-6));
#11978=CARTESIAN_POINT('Ctrl Pts',(12.9263774359968,2.16414405704371,-3.92049452767182E-6));
#11979=CARTESIAN_POINT('Ctrl Pts',(12.9083632163621,2.16518216214944,-2.15504024707585E-6));
#11980=CARTESIAN_POINT('Ctrl Pts',(12.8903762705535,2.16459816844574,-9.12104093693782E-7));
#11981=CARTESIAN_POINT('Ctrl Pts',(12.8828459063217,2.16435367528137,-3.91739933400607E-7));
#11982=CARTESIAN_POINT('Ctrl Pts',(12.8753202361859,2.1638242536466,5.87463683432524E-12));
#11983=CARTESIAN_POINT('Ctrl Pts',(12.8678148030684,2.16300527278357,2.8796409701215E-16));
#11984=CARTESIAN_POINT('',(13.2,-1.86519007666192,1.11326398357188E-16));
#11985=CARTESIAN_POINT('',(13.2,2.2,0.));
#11986=CARTESIAN_POINT('',(12.8678148030684,-2.16300527278356,1.38777878078145E-17));
#11987=CARTESIAN_POINT('Ctrl Pts',(12.8678148030684,-2.16300527278357,2.56739074444567E-16));
#11988=CARTESIAN_POINT('Ctrl Pts',(12.8854929372559,-2.16493428409685,8.24591542686399E-11));
#11989=CARTESIAN_POINT('Ctrl Pts',(12.9032520674897,-2.16521372082443,-4.52295339524789E-6));
#11990=CARTESIAN_POINT('Ctrl Pts',(12.9208958607904,-2.1639404182545,-8.68231213275745E-6));
#11991=CARTESIAN_POINT('Ctrl Pts',(12.9389012534027,-2.16264102008682,-1.29269145154966E-5));
#11992=CARTESIAN_POINT('Ctrl Pts',(12.9567880250381,-2.15972433317902,-1.67278855193166E-5));
#11993=CARTESIAN_POINT('Ctrl Pts',(12.9743443410528,-2.15524079327399,-1.78237954457702E-5));
#11994=CARTESIAN_POINT('Ctrl Pts',(12.9774431846623,-2.15444940919484,-1.80172331504298E-5));
#11995=CARTESIAN_POINT('Ctrl Pts',(12.9805316913262,-2.15360908525727,-1.81351031595367E-5));
#11996=CARTESIAN_POINT('Ctrl Pts',(12.9836086301392,-2.15271994254544,-1.81766625580856E-5));
#11997=CARTESIAN_POINT('Ctrl Pts',(13.0010041030966,-2.14769317440371,-1.84116186093898E-5));
#11998=CARTESIAN_POINT('Ctrl Pts',(13.017876958431,-2.14115457229109,-1.5854618169158E-5));
#11999=CARTESIAN_POINT('Ctrl Pts',(13.0340226638693,-2.13317744288338,-1.23136839993165E-5));
#12000=CARTESIAN_POINT('Ctrl Pts',(13.0473215411186,-2.12660684953271,-9.39709115965876E-6));
#12001=CARTESIAN_POINT('Ctrl Pts',(13.060127470267,-2.11905920305061,-5.85016632862467E-6));
#12002=CARTESIAN_POINT('Ctrl Pts',(13.0723151314263,-2.11055132433008,-4.53327195050794E-6));
#12003=CARTESIAN_POINT('Ctrl Pts',(13.0772147086919,-2.10713106111368,-4.00386555564548E-6));
#12004=CARTESIAN_POINT('Ctrl Pts',(13.0820141951123,-2.10355537352593,-3.85636210984559E-6));
#12005=CARTESIAN_POINT('Ctrl Pts',(13.0867078006727,-2.0998301147952,-3.90248451975241E-6));
#12006=CARTESIAN_POINT('Ctrl Pts',(13.1007249787291,-2.08870484782034,-4.04022639510273E-6));
#12007=CARTESIAN_POINT('Ctrl Pts',(13.1136765748478,-2.07634683247102,-5.5945154994439E-6));
#12008=CARTESIAN_POINT('Ctrl Pts',(13.1254414850725,-2.06295113861397,-5.97495381195624E-6));
#12009=CARTESIAN_POINT('Ctrl Pts',(13.1372476314214,-2.04950849272046,-6.35672556443159E-6));
#12010=CARTESIAN_POINT('Ctrl Pts',(13.1478597809499,-2.03501968083851,-5.56609061204695E-6));
#12011=CARTESIAN_POINT('Ctrl Pts',(13.1571184147632,-2.01964723728874,-4.75455255839871E-6));
#12012=CARTESIAN_POINT('Ctrl Pts',(13.158708901902,-2.01700649414547,-4.61514313115074E-6));
#12013=CARTESIAN_POINT('Ctrl Pts',(13.1602593369672,-2.01433961799121,-4.48389992381974E-6));
#12014=CARTESIAN_POINT('Ctrl Pts',(13.1617687665475,-2.01164737048868,-4.37752847101542E-6));
#12015=CARTESIAN_POINT('Ctrl Pts',(13.1632768494098,-2.00895752501823,-4.27125192317111E-6));
#12016=CARTESIAN_POINT('Ctrl Pts',(13.164742106841,-2.00624572954308,-4.19089851494128E-6));
#12017=CARTESIAN_POINT('Ctrl Pts',(13.1661638648313,-2.00351289682408,-4.15637526360595E-6));
#12018=CARTESIAN_POINT('Ctrl Pts',(13.1744716670281,-1.98754405133797,-3.95464448717833E-6));
#12019=CARTESIAN_POINT('Ctrl Pts',(13.181298057795,-1.97085874357403,-5.01850453361653E-6));
#12020=CARTESIAN_POINT('Ctrl Pts',(13.1866022393826,-1.95366776591112,-4.89891140766866E-6));
#12021=CARTESIAN_POINT('Ctrl Pts',(13.1879075264936,-1.94943729958961,-4.86948116225E-6));
#12022=CARTESIAN_POINT('Ctrl Pts',(13.1891204013114,-1.94517611908519,-4.78523710928743E-6));
#12023=CARTESIAN_POINT('Ctrl Pts',(13.1902397948733,-1.94088722910442,-4.64104147683466E-6));
#12024=CARTESIAN_POINT('Ctrl Pts',(13.1947901580114,-1.92345278286841,-4.05488258426869E-6));
#12025=CARTESIAN_POINT('Ctrl Pts',(13.1977733658442,-1.90566244769967,-2.24449026644408E-6));
#12026=CARTESIAN_POINT('Ctrl Pts',(13.1991406030032,-1.88772335428786,-9.50757284845071E-7));
#12027=CARTESIAN_POINT('Ctrl Pts',(13.1997114533543,-1.8802334044254,-4.10596478211383E-7));
#12028=CARTESIAN_POINT('Ctrl Pts',(13.2000000000958,-1.87271737110067,6.9401096738129E-12));
#12029=CARTESIAN_POINT('Ctrl Pts',(13.2,-1.86519007666192,1.81278603239576E-16));
#12030=CARTESIAN_POINT('',(0.292751161823634,-1.50665779898694,-1.38777878078145E-17));
#12031=CARTESIAN_POINT('Ctrl Pts',(12.8678148030684,-2.16300527278356,0.));
#12032=CARTESIAN_POINT('Ctrl Pts',(8.67612692265345,-1.70561506876628,0.));
#12033=CARTESIAN_POINT('Ctrl Pts',(4.48443904223854,-1.60211086545473,0.));
#12034=CARTESIAN_POINT('Ctrl Pts',(0.292751161823634,-1.50665779898694,
0.));
#12035=CARTESIAN_POINT('',(4.02814324098787E-18,-1.20714678905882,5.54818711994559E-17));
#12036=CARTESIAN_POINT('Ctrl Pts',(-2.22044604925031E-16,-1.20714678905882,
-3.98986399474666E-17));
#12037=CARTESIAN_POINT('Ctrl Pts',(2.12382277713531E-10,-1.2249878157372,
-1.35440422383976E-12));
#12038=CARTESIAN_POINT('Ctrl Pts',(0.00163882612763064,-1.24276245549475,
-1.96699749426327E-6));
#12039=CARTESIAN_POINT('Ctrl Pts',(0.00481304415265273,-1.26026068126938,
-2.66007142975038E-6));
#12040=CARTESIAN_POINT('Ctrl Pts',(0.00802873944670128,-1.27798755504872,
-3.36220171040687E-6));
#12041=CARTESIAN_POINT('Ctrl Pts',(0.0128206026099745,-1.29543230475431,
-2.69550948014298E-6));
#12042=CARTESIAN_POINT('Ctrl Pts',(0.0191320595672371,-1.31236817798419,
-4.00401478067381E-7));
#12043=CARTESIAN_POINT('Ctrl Pts',(0.0202443702650641,-1.31535290133701,
4.0809101773195E-9));
#12044=CARTESIAN_POINT('Ctrl Pts',(0.0214039964883031,-1.3183217636574,
4.5005107558061E-7));
#12045=CARTESIAN_POINT('Ctrl Pts',(0.0226107760969305,-1.32127343934773,
9.26779280916758E-7));
#12046=CARTESIAN_POINT('Ctrl Pts',(0.0294548697216842,-1.33801348419941,
3.63048130534217E-6));
#12047=CARTESIAN_POINT('Ctrl Pts',(0.0377511831708778,-1.35405403406083,
7.64722139837078E-6));
#12048=CARTESIAN_POINT('Ctrl Pts',(0.0474204318104353,-1.36917746582299,
9.03443059383348E-6));
#12049=CARTESIAN_POINT('Ctrl Pts',(0.0524109755304394,-1.37698305136733,
9.75040433665629E-6));
#12050=CARTESIAN_POINT('Ctrl Pts',(0.0577680562174045,-1.38454410063597,
9.71159147480002E-6));
#12051=CARTESIAN_POINT('Ctrl Pts',(0.0634855547170043,-1.39182806229354,
7.98761394269614E-6));
#12052=CARTESIAN_POINT('Ctrl Pts',(0.0706048733905122,-1.40089791062835,
5.84095042579577E-6));
#12053=CARTESIAN_POINT('Ctrl Pts',(0.0782829434694699,-1.40953838460506,
1.09773645972912E-6));
#12054=CARTESIAN_POINT('Ctrl Pts',(0.0864706998703675,-1.41772246232928,
-4.21049985396393E-6));
#12055=CARTESIAN_POINT('Ctrl Pts',(0.0990944981487371,-1.43034058886193,
-1.2394683793612E-5));
#12056=CARTESIAN_POINT('Ctrl Pts',(0.112816484288725,-1.44176429483685,
-2.16481703631134E-5));
#12057=CARTESIAN_POINT('Ctrl Pts',(0.127426518150943,-1.45192534842919,
-2.7562374581111E-5));
#12058=CARTESIAN_POINT('Ctrl Pts',(0.142261949549145,-1.46224316253723,
-3.35678206860622E-5));
#12059=CARTESIAN_POINT('Ctrl Pts',(0.158014355623482,-1.47125989363127,
-3.6155642403295E-5));
#12060=CARTESIAN_POINT('Ctrl Pts',(0.17449494651519,-1.47886261331763,-3.45187637154371E-5));
#12061=CARTESIAN_POINT('Ctrl Pts',(0.177115379630184,-1.48007145458801,
-3.42584981007467E-5));
#12062=CARTESIAN_POINT('Ctrl Pts',(0.179754261386328,-1.48124444832217,
-3.38986806574493E-5));
#12063=CARTESIAN_POINT('Ctrl Pts',(0.18241086941249,-1.48238102342202,-3.34441145409493E-5));
#12064=CARTESIAN_POINT('Ctrl Pts',(0.199890279181845,-1.48985922935543,
-3.04532527580594E-5));
#12065=CARTESIAN_POINT('Ctrl Pts',(0.217974246898519,-1.49569663469242,
-2.31073027206853E-5));
#12066=CARTESIAN_POINT('Ctrl Pts',(0.236436446036386,-1.49978781870256,
-1.54828395726751E-5));
#12067=CARTESIAN_POINT('Ctrl Pts',(0.253618559172887,-1.50359533838099,
-8.38702246898572E-6));
#12068=CARTESIAN_POINT('Ctrl Pts',(0.271129804961754,-1.50589051664322,
-1.1237837803371E-6));
#12069=CARTESIAN_POINT('Ctrl Pts',(0.288799387895208,-1.50654014509364,
-1.14426782679271E-7));
#12070=CARTESIAN_POINT('Ctrl Pts',(0.290115790923368,-1.5065885431154,-3.92285953074499E-8));
#12071=CARTESIAN_POINT('Ctrl Pts',(0.291433072638222,-1.50662778343727,
-2.32210426557352E-12));
#12072=CARTESIAN_POINT('Ctrl Pts',(0.292751161823634,-1.50665779898694,
2.86229373536173E-17));
#12073=CARTESIAN_POINT('',(0.,-1.5,0.));
#12074=CARTESIAN_POINT('',(0.297857995688647,-1.306435779838,0.));
#12075=CARTESIAN_POINT('Ctrl Pts',(0.200274469199585,-1.20659878095028,
-5.63785129692462E-18));
#12076=CARTESIAN_POINT('Ctrl Pts',(0.200274469233139,-1.21453676310593,
-8.71436967499621E-13));
#12077=CARTESIAN_POINT('Ctrl Pts',(0.201246859971722,-1.22243356087926,
-1.21395871814677E-6));
#12078=CARTESIAN_POINT('Ctrl Pts',(0.203115675186186,-1.23012372049816,
-1.3343733317444E-6));
#12079=CARTESIAN_POINT('Ctrl Pts',(0.204315340901654,-1.23506033529553,
-1.41167219064517E-6));
#12080=CARTESIAN_POINT('Ctrl Pts',(0.20588557457721,-1.23991201018842,-1.08820351238587E-6));
#12081=CARTESIAN_POINT('Ctrl Pts',(0.207817175189242,-1.24463217458037,
-4.7123943162984E-7));
#12082=CARTESIAN_POINT('Ctrl Pts',(0.210821635148072,-1.25197403646754,
4.8840194822981E-7));
#12083=CARTESIAN_POINT('Ctrl Pts',(0.214662962735955,-1.25891288736431,
2.34840446672759E-6));
#12084=CARTESIAN_POINT('Ctrl Pts',(0.219285851586231,-1.26528190572196,
1.77850405974346E-6));
#12085=CARTESIAN_POINT('Ctrl Pts',(0.219987799701267,-1.26624898941694,
1.69196931287913E-6));
#12086=CARTESIAN_POINT('Ctrl Pts',(0.220707854727247,-1.26720289123473,
1.54254180957111E-6));
#12087=CARTESIAN_POINT('Ctrl Pts',(0.221445913570039,-1.26814297034805,
1.31084431541716E-6));
#12088=CARTESIAN_POINT('Ctrl Pts',(0.223819423285066,-1.27116615329633,
5.65732650279818E-7));
#12089=CARTESIAN_POINT('Ctrl Pts',(0.226378993511503,-1.27404655624932,
-1.0141799309673E-6));
#12090=CARTESIAN_POINT('Ctrl Pts',(0.229108317341547,-1.27677508245113,
-2.75886047820546E-6));
#12091=CARTESIAN_POINT('Ctrl Pts',(0.234729699316268,-1.28239482161129,
-6.35224711555937E-6));
#12092=CARTESIAN_POINT('Ctrl Pts',(0.241002345945823,-1.28730653457646,
-1.03364935932408E-5));
#12093=CARTESIAN_POINT('Ctrl Pts',(0.247764463424355,-1.29145035967733,
-1.17765252099068E-5));
#12094=CARTESIAN_POINT('Ctrl Pts',(0.25202072563572,-1.29405859685204,-1.26829206064147E-5));
#12095=CARTESIAN_POINT('Ctrl Pts',(0.25647185453211,-1.29636195369988,-1.26655904667795E-5));
#12096=CARTESIAN_POINT('Ctrl Pts',(0.261083107941716,-1.29833661269995,
-1.17517412599227E-5));
#12097=CARTESIAN_POINT('Ctrl Pts',(0.268362152520619,-1.30145368947124,
-1.0309194402435E-5));
#12098=CARTESIAN_POINT('Ctrl Pts',(0.275955349537693,-1.30371808689536,
-6.50743389458559E-6));
#12099=CARTESIAN_POINT('Ctrl Pts',(0.283717840216357,-1.30505580179168,
-3.40467605837577E-6));
#12100=CARTESIAN_POINT('Ctrl Pts',(0.288379557365255,-1.3058591584372,-1.54133347766382E-6));
#12101=CARTESIAN_POINT('Ctrl Pts',(0.293102847896135,-1.30632748638856,
-3.09915230996644E-12));
#12102=CARTESIAN_POINT('Ctrl Pts',(0.297857995688647,-1.306435779838,2.90566182226115E-17));
#12103=CARTESIAN_POINT('',(0.9,-1.32024227787037,0.));
#12104=CARTESIAN_POINT('Ctrl Pts',(0.297857995688651,-1.306435779838,-5.81335652359571E-17));
#12105=CARTESIAN_POINT('Ctrl Pts',(0.498765834064439,-1.31101124067384,
-1.02216845336465E-13));
#12106=CARTESIAN_POINT('Ctrl Pts',(0.699470314209512,-1.31560060357718,
-4.73070532165219E-10));
#12107=CARTESIAN_POINT('Ctrl Pts',(0.9,-1.32024227787037,4.62320796019307E-17));
#12108=CARTESIAN_POINT('',(0.9,1.39290118819044,0.));
#12109=CARTESIAN_POINT('',(4.3,-1.41116952203211,0.));
#12110=CARTESIAN_POINT('Ctrl Pts',(1.10000000020724,-1.32489175811528,-9.82782277325449E-12));
#12111=CARTESIAN_POINT('Ctrl Pts',(2.16992692797068,-1.34987955410658,4.63225598025733E-9));
#12112=CARTESIAN_POINT('Ctrl Pts',(3.23514201430925,-1.37672428034078,3.20747301048384E-8));
#12113=CARTESIAN_POINT('Ctrl Pts',(4.3,-1.41116952203211,-8.74629427996717E-16));
#12114=CARTESIAN_POINT('',(4.3,1.48481481481482,0.));
#12115=CARTESIAN_POINT('',(8.7,-1.61160179736194,0.));
#12116=CARTESIAN_POINT('Ctrl Pts',(4.50000000001737,-1.41772989873549,-1.00870158580013E-12));
#12117=CARTESIAN_POINT('Ctrl Pts',(5.14541122039116,-1.43919849219739,1.84287460122322E-8));
#12118=CARTESIAN_POINT('Ctrl Pts',(5.79079200637672,-1.46358894290692,-2.29215846350395E-9));
#12119=CARTESIAN_POINT('Ctrl Pts',(6.43711407552466,-1.49221504703413,-7.12038357450289E-9));
#12120=CARTESIAN_POINT('Ctrl Pts',(6.48784335049204,-1.49446188584227,-7.49934689782436E-9));
#12121=CARTESIAN_POINT('Ctrl Pts',(6.5385784252675,-1.49673484630497,-7.6873350528488E-9));
#12122=CARTESIAN_POINT('Ctrl Pts',(6.58931977021612,-1.49903457911226,-7.60400982311631E-9));
#12123=CARTESIAN_POINT('Ctrl Pts',(7.29382172663923,-1.5309644828944,-6.44710735180711E-9));
#12124=CARTESIAN_POINT('Ctrl Pts',(7.99729122590638,-1.56795478022256,5.29179522587699E-9));
#12125=CARTESIAN_POINT('Ctrl Pts',(8.70000000002062,-1.61160179731554,-3.21479112539667E-13));
#12126=CARTESIAN_POINT('',(8.7,1.68851851851852,0.));
#12127=CARTESIAN_POINT('',(12.6,-1.93292824674167,0.));
#12128=CARTESIAN_POINT('',(12.8889963716306,-1.96391015057091,0.));
#12129=CARTESIAN_POINT('Ctrl Pts',(12.6000000004653,-1.93292824679067,-1.00288700954909E-16));
#12130=CARTESIAN_POINT('Ctrl Pts',(12.6963367945484,-1.94307238002033,2.28133307867826E-10));
#12131=CARTESIAN_POINT('Ctrl Pts',(12.7926686848896,-1.9533982851754,-5.07154825701885E-13));
#12132=CARTESIAN_POINT('Ctrl Pts',(12.8889963716306,-1.96391015057091,2.24786696790336E-16));
#12133=CARTESIAN_POINT('',(12.9997255308004,-1.86463850151065,-1.38777878078145E-17));
#12134=CARTESIAN_POINT('Ctrl Pts',(12.8889963716306,-1.96391015057091,5.29090660172926E-17));
#12135=CARTESIAN_POINT('Ctrl Pts',(12.8968843421745,-1.96477093437063,1.28387508960266E-11));
#12136=CARTESIAN_POINT('Ctrl Pts',(12.9048206871516,-1.96464841285931,-2.5989605143924E-6));
#12137=CARTESIAN_POINT('Ctrl Pts',(12.9126487282508,-1.9636130141884,-4.24292438262167E-6));
#12138=CARTESIAN_POINT('Ctrl Pts',(12.9176900487482,-1.96294620923983,-5.30165014054907E-6));
#12139=CARTESIAN_POINT('Ctrl Pts',(12.9226867577298,-1.96189962975099,-6.00943773338864E-6));
#12140=CARTESIAN_POINT('Ctrl Pts',(12.9275953864907,-1.96048085896027,-6.09358828708331E-6));
#12141=CARTESIAN_POINT('Ctrl Pts',(12.9352257743335,-1.95827540160737,-6.22439902734509E-6));
#12142=CARTESIAN_POINT('Ctrl Pts',(12.9425549137553,-1.95519874430406,-4.64402662178521E-6));
#12143=CARTESIAN_POINT('Ctrl Pts',(12.949425376669,-1.9513005478593,-3.15156624759025E-6));
#12144=CARTESIAN_POINT('Ctrl Pts',(12.9520760960011,-1.94979656991686,-2.57575445499556E-6));
#12145=CARTESIAN_POINT('Ctrl Pts',(12.9546583803074,-1.94816978416017,-2.04880625960079E-6));
#12146=CARTESIAN_POINT('Ctrl Pts',(12.9571622133441,-1.9464211898676,-1.82278374303809E-6));
#12147=CARTESIAN_POINT('Ctrl Pts',(12.9587955877505,-1.9452804951316,-1.67533805140214E-6));
#12148=CARTESIAN_POINT('Ctrl Pts',(12.9603955609302,-1.94408794089591,-1.65796127395168E-6));
#12149=CARTESIAN_POINT('Ctrl Pts',(12.9619602112942,-1.94284549575182,-1.70649031798611E-6));
#12150=CARTESIAN_POINT('Ctrl Pts',(12.9681665721336,-1.93791719798967,-1.89898620422551E-6));
#12151=CARTESIAN_POINT('Ctrl Pts',(12.9737470546445,-1.93226498850035,-2.8025064238469E-6));
#12152=CARTESIAN_POINT('Ctrl Pts',(12.9786034821464,-1.926037248212,-2.79230211737029E-6));
#12153=CARTESIAN_POINT('Ctrl Pts',(12.9817011960737,-1.92206483066456,-2.78579321297956E-6));
#12154=CARTESIAN_POINT('Ctrl Pts',(12.9845038017717,-1.91785723501915,-2.48811564693169E-6));
#12155=CARTESIAN_POINT('Ctrl Pts',(12.9869771252785,-1.91344616543364,-2.2918341012218E-6));
#12156=CARTESIAN_POINT('Ctrl Pts',(12.9874796596041,-1.91254991636901,-2.25195326317628E-6));
#12157=CARTESIAN_POINT('Ctrl Pts',(12.9879679417815,-1.9116463809131,-2.21866365029432E-6));
#12158=CARTESIAN_POINT('Ctrl Pts',(12.98844174868,-1.91073586520696,-2.19841011183313E-6));
#12159=CARTESIAN_POINT('Ctrl Pts',(12.9918929665356,-1.9041036526468,-2.05088297829219E-6));
#12160=CARTESIAN_POINT('Ctrl Pts',(12.9945793344589,-1.89710244289626,-2.35789128083535E-6));
#12161=CARTESIAN_POINT('Ctrl Pts',(12.9964698429198,-1.88986530397042,-1.93853625224654E-6));
#12162=CARTESIAN_POINT('Ctrl Pts',(12.9984668213505,-1.88222058265133,-1.49556391743615E-6));
#12163=CARTESIAN_POINT('Ctrl Pts',(12.9995610814633,-1.87437060764114,-2.4459616079733E-7));
#12164=CARTESIAN_POINT('Ctrl Pts',(12.9997084424383,-1.86646992060833,-2.60951667192209E-8));
#12165=CARTESIAN_POINT('Ctrl Pts',(12.9997198235207,-1.86585972940924,-9.21975031242219E-9));
#12166=CARTESIAN_POINT('Ctrl Pts',(12.9997255308031,-1.86524923282631,2.14479566203628E-13));
#12167=CARTESIAN_POINT('Ctrl Pts',(12.9997255308004,-1.86463850151065,-9.54097911787244E-18));
#12168=CARTESIAN_POINT('',(12.9997255308004,1.86463850151064,1.38777878078145E-17));
#12169=CARTESIAN_POINT('',(12.9997255308004,1.1,0.));
#12170=CARTESIAN_POINT('',(12.8889963716306,1.96391015057091,0.));
#12171=CARTESIAN_POINT('Ctrl Pts',(12.9997255308004,1.86463850151065,-9.97465998686664E-18));
#12172=CARTESIAN_POINT('Ctrl Pts',(12.9997255309996,1.87257112921612,1.42345874390777E-11));
#12173=CARTESIAN_POINT('Ctrl Pts',(12.9987425107347,1.88044501776258,-2.76622459581243E-6));
#12174=CARTESIAN_POINT('Ctrl Pts',(12.9968635501128,1.8881121101061,-4.50602169498049E-6));
#12175=CARTESIAN_POINT('Ctrl Pts',(12.9956551765012,1.89304287446485,-5.62489820561454E-6));
#12176=CARTESIAN_POINT('Ctrl Pts',(12.994075066483,1.89788828888188,-6.37205869803057E-6));
#12177=CARTESIAN_POINT('Ctrl Pts',(12.9921354490207,1.90260616696402,-6.45954116508302E-6));
#12178=CARTESIAN_POINT('Ctrl Pts',(12.9891151690915,1.90995262200289,-6.59576469602218E-6));
#12179=CARTESIAN_POINT('Ctrl Pts',(12.9852608829945,1.91690476599405,-4.92589918404109E-6));
#12180=CARTESIAN_POINT('Ctrl Pts',(12.9806393828366,1.92331154882078,-3.3382766296878E-6));
#12181=CARTESIAN_POINT('Ctrl Pts',(12.9788533632605,1.92578750666072,-2.72472586378502E-6));
#12182=CARTESIAN_POINT('Ctrl Pts',(12.9769522584487,1.92818179997524,-2.1610482659023E-6));
#12183=CARTESIAN_POINT('Ctrl Pts',(12.9749381758772,1.93048453804291,-1.90960564360578E-6));
#12184=CARTESIAN_POINT('Ctrl Pts',(12.9736352090466,1.93197424425657,-1.74694031832382E-6));
#12185=CARTESIAN_POINT('Ctrl Pts',(12.9722849384098,1.93342561524533,-1.71698229815602E-6));
#12186=CARTESIAN_POINT('Ctrl Pts',(12.9708894910408,1.9348369915754,-1.75552529092739E-6));
#12187=CARTESIAN_POINT('Ctrl Pts',(12.9653179015399,1.94047218048862,-1.90941553332435E-6));
#12188=CARTESIAN_POINT('Ctrl Pts',(12.9590944588136,1.94540670303376,-2.83773366290493E-6));
#12189=CARTESIAN_POINT('Ctrl Pts',(12.9523775255978,1.94955941520082,-2.8574013135715E-6));
#12190=CARTESIAN_POINT('Ctrl Pts',(12.9480923984168,1.95220867479748,-2.86994846593266E-6));
#12191=CARTESIAN_POINT('Ctrl Pts',(12.9436054681019,1.95453912223498,-2.59559485065602E-6));
#12192=CARTESIAN_POINT('Ctrl Pts',(12.9389519978263,1.95652032281755,-2.39773084743613E-6));
#12193=CARTESIAN_POINT('Ctrl Pts',(12.9379934875219,1.95692840561619,-2.35697530915642E-6));
#12194=CARTESIAN_POINT('Ctrl Pts',(12.9370291206935,1.95732112306527,-2.32193094846859E-6));
#12195=CARTESIAN_POINT('Ctrl Pts',(12.9360592398442,1.95769827921557,-2.29894501965994E-6));
#12196=CARTESIAN_POINT('Ctrl Pts',(12.929096105975,1.96040602292032,-2.13392052256244E-6));
#12197=CARTESIAN_POINT('Ctrl Pts',(12.9218497638689,1.96231496375013,-2.36509085467933E-6));
#12198=CARTESIAN_POINT('Ctrl Pts',(12.9144555496645,1.96340894166242,-1.92146179377921E-6));
#12199=CARTESIAN_POINT('Ctrl Pts',(12.9066371708262,1.96456567495722,-1.45238421961943E-6));
#12200=CARTESIAN_POINT('Ctrl Pts',(12.8987125532455,1.96480297730229,-2.37321368026999E-7));
#12201=CARTESIAN_POINT('Ctrl Pts',(12.8908401755085,1.96409377829808,-2.55627471131237E-8));
#12202=CARTESIAN_POINT('Ctrl Pts',(12.89022523009,1.96403837970149,-9.02136684357828E-9));
#12203=CARTESIAN_POINT('Ctrl Pts',(12.8896106033158,1.96397717928728,1.9621770460073E-13));
#12204=CARTESIAN_POINT('Ctrl Pts',(12.8889963716306,1.96391015057091,-3.29597460435593E-17));
#12205=CARTESIAN_POINT('',(12.6,1.93292824674167,0.));
#12206=CARTESIAN_POINT('Ctrl Pts',(12.8889963716306,1.96391015057091,8.95144418658345E-17));
#12207=CARTESIAN_POINT('Ctrl Pts',(12.7926686852738,1.95339828521733,-5.07275478770449E-13));
#12208=CARTESIAN_POINT('Ctrl Pts',(12.6963367949308,1.94307238006059,2.28132759158623E-10));
#12209=CARTESIAN_POINT('Ctrl Pts',(12.6000000004652,1.93292824679066,-1.5019386425618E-16));
#12210=CARTESIAN_POINT('',(12.6,-1.99376954809806,0.));
#12211=CARTESIAN_POINT('Origin',(11.2,0.,0.));
#12212=CARTESIAN_POINT('',(10.8,-4.89858719658942E-17,0.7));
#12213=CARTESIAN_POINT('Origin',(11.2,0.,0.7));
#12214=CARTESIAN_POINT('',(10.8,-4.89858719658942E-17,0.));
#12215=CARTESIAN_POINT('Origin',(2.,0.,0.));
#12216=CARTESIAN_POINT('',(1.6,-4.89858719658941E-17,0.));
#12217=CARTESIAN_POINT('Origin',(12.6,-1.99376954809806,0.));
#12218=CARTESIAN_POINT('',(12.6,-1.90428042248893,0.60470250816874));
#12219=CARTESIAN_POINT('Ctrl Pts',(12.6,-1.93292824674167,0.));
#12220=CARTESIAN_POINT('Ctrl Pts',(12.6,-1.92814118331811,0.100975624959503));
#12221=CARTESIAN_POINT('Ctrl Pts',(12.6,-1.9233557423333,0.20195205683881));
#12222=CARTESIAN_POINT('Ctrl Pts',(12.6,-1.91380649287245,0.40351907263528));
#12223=CARTESIAN_POINT('Ctrl Pts',(12.6,-1.90904260275794,0.504111110768618));
#12224=CARTESIAN_POINT('Ctrl Pts',(12.6,-1.90428042248893,0.60470250816874));
#12225=CARTESIAN_POINT('',(12.6,1.90428042248893,0.60470250816874));
#12226=CARTESIAN_POINT('Ctrl Pts',(12.6,1.90428042248893,0.60470250816874));
#12227=CARTESIAN_POINT('Ctrl Pts',(12.6,1.90904310126474,0.504100580823831));
#12228=CARTESIAN_POINT('Ctrl Pts',(12.6,1.91380749024866,0.403498012513773));
#12229=CARTESIAN_POINT('Ctrl Pts',(12.6,1.92335674041114,0.201930996640285));
#12230=CARTESIAN_POINT('Ctrl Pts',(12.6,1.92814168252712,0.100965094925255));
#12231=CARTESIAN_POINT('Ctrl Pts',(12.6,1.93292824674167,0.));
#12232=CARTESIAN_POINT('',(12.6,1.80383022254432,0.7));
#12233=CARTESIAN_POINT('Ctrl Pts',(12.6,1.80383022254432,0.7));
#12234=CARTESIAN_POINT('Ctrl Pts',(12.6,1.81177675668304,0.7));
#12235=CARTESIAN_POINT('Ctrl Pts',(12.6000021803669,1.81966206665253,0.699006623620781));
#12236=CARTESIAN_POINT('Ctrl Pts',(12.6000040789681,1.8273451885609,0.69711902809518));
#12237=CARTESIAN_POINT('Ctrl Pts',(12.6000050614635,1.8313210797205,0.696142227980247));
#12238=CARTESIAN_POINT('Ctrl Pts',(12.6000059683507,1.83524283435206,0.694925046992878));
#12239=CARTESIAN_POINT('Ctrl Pts',(12.6000066021136,1.83908960013903,0.693475985595303));
#12240=CARTESIAN_POINT('Ctrl Pts',(12.6000078338507,1.84656590463324,0.690659691378536));
#12241=CARTESIAN_POINT('Ctrl Pts',(12.6000078244032,1.85367932786264,0.687000939374075));
#12242=CARTESIAN_POINT('Ctrl Pts',(12.6000065509639,1.86028396908448,0.682580904467878));
#12243=CARTESIAN_POINT('Ctrl Pts',(12.600005740321,1.86448833536622,0.679767209507086));
#12244=CARTESIAN_POINT('Ctrl Pts',(12.6000044390918,1.86848632867783,0.676643963831362));
#12245=CARTESIAN_POINT('Ctrl Pts',(12.6000033339006,1.8722338275817,0.673223162566374));
#12246=CARTESIAN_POINT('Ctrl Pts',(12.6000024442799,1.87525036668517,0.670469597843409));
#12247=CARTESIAN_POINT('Ctrl Pts',(12.600001679327,1.8780865799519,0.667539409933064));
#12248=CARTESIAN_POINT('Ctrl Pts',(12.600001676908,1.88072259809992,0.664442334323256));
#12249=CARTESIAN_POINT('Ctrl Pts',(12.6000016722164,1.88583495965423,0.658435786041233));
#12250=CARTESIAN_POINT('Ctrl Pts',(12.6000042182276,1.89019731592974,0.651802923597933));
#12251=CARTESIAN_POINT('Ctrl Pts',(12.6000050838539,1.89374834224248,0.644708005294394));
#12252=CARTESIAN_POINT('Ctrl Pts',(12.60000518898,1.89417959722901,0.643846361750254));
#12253=CARTESIAN_POINT('Ctrl Pts',(12.6000052753339,1.8945988291305,0.642977876839351));
#12254=CARTESIAN_POINT('Ctrl Pts',(12.6000053405091,1.89500587920016,0.642102827114796));
#12255=CARTESIAN_POINT('Ctrl Pts',(12.6000058761205,1.89835102950234,0.634911640898031));
#12256=CARTESIAN_POINT('Ctrl Pts',(12.6000044960414,1.90083797337412,0.627363460372113));
#12257=CARTESIAN_POINT('Ctrl Pts',(12.6000025707297,1.90241244660326,0.619625605651968));
#12258=CARTESIAN_POINT('Ctrl Pts',(12.6000013488022,1.90341170938816,0.614714661398562));
#12259=CARTESIAN_POINT('Ctrl Pts',(12.5999999979477,1.90404256918024,0.609726685483646));
#12260=CARTESIAN_POINT('Ctrl Pts',(12.6000000000242,1.90428042250026,0.604702508168697));
#12261=CARTESIAN_POINT('',(12.6,-1.8038302225439,0.7));
#12262=CARTESIAN_POINT('',(12.6,-0.996884774049031,0.7));
#12263=CARTESIAN_POINT('Ctrl Pts',(12.6000000000242,-1.90428042250026,0.604702508168697));
#12264=CARTESIAN_POINT('Ctrl Pts',(12.5999999967566,-1.90390613686288,0.612608546261599));
#12265=CARTESIAN_POINT('Ctrl Pts',(12.6000030637542,-1.90256112855112,0.620429349781532));
#12266=CARTESIAN_POINT('Ctrl Pts',(12.6000044618611,-1.90032851942705,0.628004813168584));
#12267=CARTESIAN_POINT('Ctrl Pts',(12.6000051410147,-1.89924399238468,0.63168472059761));
#12268=CARTESIAN_POINT('Ctrl Pts',(12.6000055125137,-1.89794920179963,0.635306724151721));
#12269=CARTESIAN_POINT('Ctrl Pts',(12.6000054780251,-1.8964494555225,0.638851301608537));
#12270=CARTESIAN_POINT('Ctrl Pts',(12.6000054068101,-1.89335265044601,0.64617044994032));
#12271=CARTESIAN_POINT('Ctrl Pts',(12.6000033360581,-1.88942004582711,0.653077891556402));
#12272=CARTESIAN_POINT('Ctrl Pts',(12.6000021947065,-1.88472046879005,0.659412676045522));
#12273=CARTESIAN_POINT('Ctrl Pts',(12.6000018847951,-1.88344439178375,0.661132761228218));
#12274=CARTESIAN_POINT('Ctrl Pts',(12.6000016718208,-1.88211149822114,0.662810505670431));
#12275=CARTESIAN_POINT('Ctrl Pts',(12.6000016744967,-1.88072259784382,0.664442334323417));
#12276=CARTESIAN_POINT('Ctrl Pts',(12.6000016781594,-1.87882150924004,0.666675936463772));
#12277=CARTESIAN_POINT('Ctrl Pts',(12.6000020841502,-1.87681550570489,0.668823545630641));
#12278=CARTESIAN_POINT('Ctrl Pts',(12.6000026366798,-1.87471194035196,0.670881441794774));
#12279=CARTESIAN_POINT('Ctrl Pts',(12.6000041308351,-1.86902346102148,0.676446422116204));
#12280=CARTESIAN_POINT('Ctrl Pts',(12.600006461375,-1.86269053299793,0.681293522350018));
#12281=CARTESIAN_POINT('Ctrl Pts',(12.6000072160154,-1.85587841208407,0.685370830723365));
#12282=CARTESIAN_POINT('Ctrl Pts',(12.6000077023835,-1.85148797774957,0.687998669380522));
#12283=CARTESIAN_POINT('Ctrl Pts',(12.6000076405209,-1.84689749427555,0.690306084934615));
#12284=CARTESIAN_POINT('Ctrl Pts',(12.6000070464578,-1.84214500723865,0.692269637845719));
#12285=CARTESIAN_POINT('Ctrl Pts',(12.6000061272438,-1.8347913233911,0.69530790964196));
#12286=CARTESIAN_POINT('Ctrl Pts',(12.6000039197963,-1.82713360831075,0.697490862850871));
#12287=CARTESIAN_POINT('Ctrl Pts',(12.6000021173902,-1.81932000848244,0.698749700991972));
#12288=CARTESIAN_POINT('Ctrl Pts',(12.6000009388424,-1.81421089282246,0.699572823470905));
#12289=CARTESIAN_POINT('Ctrl Pts',(12.6,-1.80903450780073,0.7));
#12290=CARTESIAN_POINT('Ctrl Pts',(12.6,-1.80383022254432,0.7));
#12291=CARTESIAN_POINT('Ctrl Pts',(12.4277899437912,-1.91498765980368,8.1061082099175E-6));
#12292=CARTESIAN_POINT('Ctrl Pts',(12.4185093097394,-1.90440735427916,0.201956437811591));
#12293=CARTESIAN_POINT('Ctrl Pts',(12.4092288296506,-1.89382707230216,0.403904777849331));
#12294=CARTESIAN_POINT('Ctrl Pts',(12.3999485057213,-1.88324681432718,0.605853126346544));
#12295=CARTESIAN_POINT('Ctrl Pts',(11.2514531524596,-1.79377193015415,-0.000335869645892519));
#12296=CARTESIAN_POINT('Ctrl Pts',(11.2440495594319,-1.78319067664719,0.201611894978303));
#12297=CARTESIAN_POINT('Ctrl Pts',(11.2366461029568,-1.77260943823668,0.403559665746509));
#12298=CARTESIAN_POINT('Ctrl Pts',(11.2292427771396,-1.76202821861547,0.605507441576721));
#12299=CARTESIAN_POINT('Ctrl Pts',(10.0755218259154,-1.69940246002113,-0.00057195363688788));
#12300=CARTESIAN_POINT('Ctrl Pts',(10.0699958446785,-1.68882059084335,0.201375418496625));
#12301=CARTESIAN_POINT('Ctrl Pts',(10.0644699805481,-1.67823873210945,0.403322794723726));
#12302=CARTESIAN_POINT('Ctrl Pts',(10.0589442279885,-1.66765688783508,0.605270174140068));
#12303=CARTESIAN_POINT('Ctrl Pts',(8.90001330805802,-1.62424530699552,-0.000736768987564917));
#12304=CARTESIAN_POINT('Ctrl Pts',(8.89636559238287,-1.61366301035882,0.201210329036737));
#12305=CARTESIAN_POINT('Ctrl Pts',(8.89271797406169,-1.60308072296431,0.403157429313698));
#12306=CARTESIAN_POINT('Ctrl Pts',(8.88907045450167,-1.59249844499155,0.605104531878289));
#12307=CARTESIAN_POINT('Ctrl Pts',(8.9000000009702,-1.5932011715731,0.605106081469384));
#12308=CARTESIAN_POINT('Ctrl Pts',(10.0684994345535,-1.66840362346204,0.605023135335662));
#12309=CARTESIAN_POINT('Ctrl Pts',(11.2356615742313,-1.76272273105624,0.604904457271936));
#12310=CARTESIAN_POINT('Ctrl Pts',(12.4,-1.8833055216247,0.604732563714112));
#12311=CARTESIAN_POINT('Ctrl Pts',(12.8889963716306,-1.96391015057091,2.25514051876985E-16));
#12312=CARTESIAN_POINT('Ctrl Pts',(12.8789974396847,-1.95334878321431,0.201594505485581));
#12313=CARTESIAN_POINT('Ctrl Pts',(12.8689986695879,-1.94278744208821,0.403189020401051));
#12314=CARTESIAN_POINT('Ctrl Pts',(12.8590000636394,-1.93222612769726,0.604783544887274));
#12315=CARTESIAN_POINT('Ctrl Pts',(12.792662965057,-1.95339909479377,-3.05216148415599E-5));
#12316=CARTESIAN_POINT('Ctrl Pts',(12.7828174539371,-1.94283764251598,0.201563933758495));
#12317=CARTESIAN_POINT('Ctrl Pts',(12.7729721028852,-1.93227621586528,0.403158398317997));
#12318=CARTESIAN_POINT('Ctrl Pts',(12.7631269141758,-1.92171481533493,0.604752872200892));
#12319=CARTESIAN_POINT('Ctrl Pts',(12.6963322449993,-1.94307475200589,-6.02899321993968E-5));
#12320=CARTESIAN_POINT('Ctrl Pts',(12.6866401583647,-1.93251321719056,0.201534116532542));
#12321=CARTESIAN_POINT('Ctrl Pts',(12.6769482300299,-1.92195170741534,0.403128531945268));
#12322=CARTESIAN_POINT('Ctrl Pts',(12.6672564622455,-1.91139022316239,0.604722956439736));
#12323=CARTESIAN_POINT('Ctrl Pts',(12.6000042264769,-1.9329329264796,-8.93242901516475E-5));
#12324=CARTESIAN_POINT('Ctrl Pts',(12.5904655680581,-1.92237131142302,0.201505034443145));
#12325=CARTESIAN_POINT('Ctrl Pts',(12.5809270661843,-1.91180972083551,0.403099401891705));
#12326=CARTESIAN_POINT('Ctrl Pts',(12.5713887230828,-1.90124815518829,0.604693778185974));
#12327=CARTESIAN_POINT('',(12.8572578715866,-1.93204080633595,0.60466226999893));
#12328=CARTESIAN_POINT('Ctrl Pts',(12.6000000000242,-1.90428042250026,0.604702508168697));
#12329=CARTESIAN_POINT('Ctrl Pts',(12.6857696261193,-1.91338852735451,0.604689390578107));
#12330=CARTESIAN_POINT('Ctrl Pts',(12.7715225733429,-1.92264108900731,0.604675979983877));
#12331=CARTESIAN_POINT('Ctrl Pts',(12.8572578715866,-1.93204080633595,0.60466226999893));
#12332=CARTESIAN_POINT('Ctrl Pts',(12.8572578715866,-1.93204080633595,0.604662269998931));
#12333=CARTESIAN_POINT('Ctrl Pts',(12.867837444884,-1.94266422047353,0.403108198925376));
#12334=CARTESIAN_POINT('Ctrl Pts',(12.8784169445746,-1.95328733374019,0.201554108835025));
#12335=CARTESIAN_POINT('Ctrl Pts',(12.8889963716306,-1.96391015057091,-1.13624387676481E-16));
#12336=CARTESIAN_POINT('Ctrl Pts',(12.4102890066107,-1.7839488953552,0.7));
#12337=CARTESIAN_POINT('Ctrl Pts',(11.2423261062923,-1.6629989551888,0.7));
#12338=CARTESIAN_POINT('Ctrl Pts',(10.0717272052363,-1.56846077660453,0.7));
#12339=CARTESIAN_POINT('Ctrl Pts',(8.89999999999993,-1.49312521822106,0.7));
#12340=CARTESIAN_POINT('Ctrl Pts',(12.4072999778185,-1.81281269415102,0.7));
#12341=CARTESIAN_POINT('Ctrl Pts',(11.2397765858669,-1.69187462084457,0.699998757165067));
#12342=CARTESIAN_POINT('Ctrl Pts',(10.0695527221263,-1.59734372851255,0.700000594792869));
#12343=CARTESIAN_POINT('Ctrl Pts',(8.89814271406455,-1.52201240649035,0.7));
#12344=CARTESIAN_POINT('Ctrl Pts',(12.4021203845267,-1.86282985658401,0.676448561733929));
#12345=CARTESIAN_POINT('Ctrl Pts',(11.2353531757414,-1.74191593276004,0.676505236381959));
#12346=CARTESIAN_POINT('Ctrl Pts',(10.0657879841113,-1.64739716848489,0.676543604639643));
#12347=CARTESIAN_POINT('Ctrl Pts',(8.89492397206972,-1.57207492202614,0.676570833338327));
#12348=CARTESIAN_POINT('Ctrl Pts',(12.400106093269,-1.88228102337346,0.626471792264191));
#12349=CARTESIAN_POINT('Ctrl Pts',(11.2336287644773,-1.76143987438699,0.626617923584012));
#12350=CARTESIAN_POINT('Ctrl Pts',(10.0643137348541,-1.66697079985262,0.626717999675944));
#12351=CARTESIAN_POINT('Ctrl Pts',(8.89366330605793,-1.59168261717615,0.626788336025017));
#12352=CARTESIAN_POINT('Ctrl Pts',(12.4,-1.8833055216247,0.604732563714112));
#12353=CARTESIAN_POINT('Ctrl Pts',(11.2335332423564,-1.7625023138725,0.604904771481731));
#12354=CARTESIAN_POINT('Ctrl Pts',(10.0642324382527,-1.66805889332185,0.605023569028795));
#12355=CARTESIAN_POINT('Ctrl Pts',(8.89359217382714,-1.59278896817116,0.605106535971077));
#12356=CARTESIAN_POINT('Ctrl Pts',(12.400000003046,-1.78288409409898,0.7));
#12357=CARTESIAN_POINT('Ctrl Pts',(11.235451325406,-1.66244391065713,0.7));
#12358=CARTESIAN_POINT('Ctrl Pts',(10.0682865064676,-1.56823955876321,0.7));
#12359=CARTESIAN_POINT('Ctrl Pts',(8.89999999999993,-1.49312521822106,0.7));
#12360=CARTESIAN_POINT('Ctrl Pts',(12.8681436286308,-1.83274446434879,0.7));
#12361=CARTESIAN_POINT('Ctrl Pts',(12.7787800350189,-1.82294762441299,0.7));
#12362=CARTESIAN_POINT('Ctrl Pts',(12.6893984576578,-1.8133105623702,0.7));
#12363=CARTESIAN_POINT('Ctrl Pts',(12.6,-1.80383022254431,0.7));
#12364=CARTESIAN_POINT('Ctrl Pts',(12.8649798835675,-1.86160311979107,0.7));
#12365=CARTESIAN_POINT('Ctrl Pts',(12.7756511334299,-1.85180730951691,0.699999896874207));
#12366=CARTESIAN_POINT('Ctrl Pts',(12.686303642571,-1.84217134991284,0.700000098415946));
#12367=CARTESIAN_POINT('Ctrl Pts',(12.5969393303221,-1.83269196733649,0.7));
#12368=CARTESIAN_POINT('Ctrl Pts',(12.8594976525144,-1.91161025179704,0.676425356750174));
#12369=CARTESIAN_POINT('Ctrl Pts',(12.7702288461641,-1.90181652272411,0.676430055978541));
#12370=CARTESIAN_POINT('Ctrl Pts',(12.6809412203008,-1.89218243450198,0.676434576658958));
#12371=CARTESIAN_POINT('Ctrl Pts',(12.5916356538948,-1.88270499442535,0.67643906321291));
#12372=CARTESIAN_POINT('Ctrl Pts',(12.8573684983393,-1.93103170500986,0.626412260100396));
#12373=CARTESIAN_POINT('Ctrl Pts',(12.7681225846323,-1.92124403769089,0.626424372515079));
#12374=CARTESIAN_POINT('Ctrl Pts',(12.6788572782757,-1.91161594713487,0.626436135819418));
#12375=CARTESIAN_POINT('Ctrl Pts',(12.5895741974899,-1.90214427893475,0.626447702441804));
#12376=CARTESIAN_POINT('Ctrl Pts',(12.8572578715866,-1.93204080633595,0.60466226999893));
#12377=CARTESIAN_POINT('Ctrl Pts',(12.7680127446979,-1.92225628370762,0.604676541242762));
#12378=CARTESIAN_POINT('Ctrl Pts',(12.6787484942245,-1.91263121188365,0.60469048808123));
#12379=CARTESIAN_POINT('Ctrl Pts',(12.5894662143615,-1.9031625467727,0.604704117718382));
#12380=CARTESIAN_POINT('',(12.8681436286308,-1.83274446434879,0.7));
#12381=CARTESIAN_POINT('Ctrl Pts',(12.8681436286308,-1.83274446434879,0.7));
#12382=CARTESIAN_POINT('Ctrl Pts',(12.7787800350189,-1.82294762441299,0.7));
#12383=CARTESIAN_POINT('Ctrl Pts',(12.6893984576578,-1.8133105623702,0.7));
#12384=CARTESIAN_POINT('Ctrl Pts',(12.6,-1.80383022254431,0.7));
#12385=CARTESIAN_POINT('Origin',(12.8681436286308,-1.83274446434879,0.6));
#12386=CARTESIAN_POINT('Origin',(6.87409734069396,-2.22251806091942E-16,
0.7));
#12387=CARTESIAN_POINT('Ctrl Pts',(8.9,1.49312521822106,0.7));
#12388=CARTESIAN_POINT('Ctrl Pts',(10.0682865064677,1.56823955876321,0.7));
#12389=CARTESIAN_POINT('Ctrl Pts',(11.2354513254061,1.66244391065714,0.7));
#12390=CARTESIAN_POINT('Ctrl Pts',(12.4000000030461,1.78288409409899,0.7));
#12391=CARTESIAN_POINT('Origin',(6.87409734069396,-2.22251806091942E-16,
0.7));
#12392=CARTESIAN_POINT('',(12.8681436286308,1.83274446434879,0.7));
#12393=CARTESIAN_POINT('Ctrl Pts',(12.6,1.80383022254432,0.7));
#12394=CARTESIAN_POINT('Ctrl Pts',(12.6893984576578,1.8133105623702,0.7));
#12395=CARTESIAN_POINT('Ctrl Pts',(12.7787800350189,1.82294762441299,0.7));
#12396=CARTESIAN_POINT('Ctrl Pts',(12.8681436286308,1.83274446434879,0.7));
#12397=CARTESIAN_POINT('',(12.8681436286308,1.1,0.7));
#12398=CARTESIAN_POINT('Ctrl Pts',(8.9,1.49312521822106,0.7));
#12399=CARTESIAN_POINT('Ctrl Pts',(10.0717272052363,1.56846077660453,0.7));
#12400=CARTESIAN_POINT('Ctrl Pts',(11.2423261062923,1.6629989551888,0.7));
#12401=CARTESIAN_POINT('Ctrl Pts',(12.4102890066107,1.7839488953552,0.7));
#12402=CARTESIAN_POINT('Ctrl Pts',(8.89814271406461,1.52201240649035,0.7));
#12403=CARTESIAN_POINT('Ctrl Pts',(10.0695527221263,1.59734372851256,0.700000594792869));
#12404=CARTESIAN_POINT('Ctrl Pts',(11.2397765858669,1.69187462084457,0.699998757165067));
#12405=CARTESIAN_POINT('Ctrl Pts',(12.4072999778185,1.81281269415102,0.7));
#12406=CARTESIAN_POINT('Ctrl Pts',(8.89492397206979,1.57207492202615,0.676570833338327));
#12407=CARTESIAN_POINT('Ctrl Pts',(10.0657879841114,1.64739716848489,0.676543604639644));
#12408=CARTESIAN_POINT('Ctrl Pts',(11.2353531757414,1.74191593276004,0.676505236381959));
#12409=CARTESIAN_POINT('Ctrl Pts',(12.4021203845267,1.86282985658401,0.676448561733929));
#12410=CARTESIAN_POINT('Ctrl Pts',(8.89366330605799,1.59168261717616,0.626788336025017));
#12411=CARTESIAN_POINT('Ctrl Pts',(10.0643137348542,1.66697079985262,0.626717999675944));
#12412=CARTESIAN_POINT('Ctrl Pts',(11.2336287644773,1.761439874387,0.626617923584012));
#12413=CARTESIAN_POINT('Ctrl Pts',(12.400106093269,1.88228102337346,0.626471792264191));
#12414=CARTESIAN_POINT('Ctrl Pts',(8.89359217382721,1.59278896817116,0.605106535971077));
#12415=CARTESIAN_POINT('Ctrl Pts',(10.0642324382527,1.66805889332185,0.605023569028795));
#12416=CARTESIAN_POINT('Ctrl Pts',(11.2335332423565,1.7625023138725,0.604904771481731));
#12417=CARTESIAN_POINT('Ctrl Pts',(12.4,1.8833055216247,0.604732563714112));
#12418=CARTESIAN_POINT('Ctrl Pts',(12.4,1.8833055216247,0.604732563714112));
#12419=CARTESIAN_POINT('Ctrl Pts',(11.2356615742313,1.76272273105624,0.604904457271936));
#12420=CARTESIAN_POINT('Ctrl Pts',(10.0684994345535,1.66840362346204,0.605023135335662));
#12421=CARTESIAN_POINT('Ctrl Pts',(8.90000000097019,1.5932011715731,0.605106081469384));
#12422=CARTESIAN_POINT('Ctrl Pts',(8.90001330805765,1.62424530699444,-0.000736768966955875));
#12423=CARTESIAN_POINT('Ctrl Pts',(8.89636559238262,1.6136630103581,0.201210329050476));
#12424=CARTESIAN_POINT('Ctrl Pts',(8.89271797406156,1.60308072296395,0.403157429320568));
#12425=CARTESIAN_POINT('Ctrl Pts',(8.88907045450167,1.59249844499155,0.605104531878289));
#12426=CARTESIAN_POINT('Ctrl Pts',(10.0755218259151,1.69940246002007,-0.000571953616278766));
#12427=CARTESIAN_POINT('Ctrl Pts',(10.0699958446785,1.68882059084265,0.201375418510364));
#12428=CARTESIAN_POINT('Ctrl Pts',(10.0644699805483,1.67823873210911,0.403322794730596));
#12429=CARTESIAN_POINT('Ctrl Pts',(10.0589442279888,1.6676568878351,0.605270174140069));
#12430=CARTESIAN_POINT('Ctrl Pts',(11.2514531524595,1.79377193015312,-0.000335869625283423));
#12431=CARTESIAN_POINT('Ctrl Pts',(11.244049559432,1.78319067664652,0.201611894992042));
#12432=CARTESIAN_POINT('Ctrl Pts',(11.2366461029572,1.77260943823637,0.403559665753379));
#12433=CARTESIAN_POINT('Ctrl Pts',(11.2292427771402,1.76202821861552,0.605507441576721));
#12434=CARTESIAN_POINT('Ctrl Pts',(12.4277899437912,1.9149876598027,8.10612881915578E-6));
#12435=CARTESIAN_POINT('Ctrl Pts',(12.4185093097397,1.90440735427854,0.201956437825331));
#12436=CARTESIAN_POINT('Ctrl Pts',(12.4092288296513,1.89382707230189,0.403904777856201));
#12437=CARTESIAN_POINT('Ctrl Pts',(12.3999485057223,1.88324681432728,0.605853126346545));
#12438=CARTESIAN_POINT('Ctrl Pts',(12.6000042264759,1.9329329264795,-8.93242901520291E-5));
#12439=CARTESIAN_POINT('Ctrl Pts',(12.5904655680574,1.92237131142328,0.201505034436202));
#12440=CARTESIAN_POINT('Ctrl Pts',(12.580927066184,1.91180972083614,0.403099401877819));
#12441=CARTESIAN_POINT('Ctrl Pts',(12.5713887230828,1.90124815518927,0.604693778165146));
#12442=CARTESIAN_POINT('Ctrl Pts',(12.6963322449987,1.94307475200582,-6.02899321996874E-5));
#12443=CARTESIAN_POINT('Ctrl Pts',(12.6866401583644,1.93251321719085,0.201534116525599));
#12444=CARTESIAN_POINT('Ctrl Pts',(12.6769482300299,1.921951707416,0.403128531931383));
#12445=CARTESIAN_POINT('Ctrl Pts',(12.6672564622458,1.91139022316341,0.604722956418908));
#12446=CARTESIAN_POINT('Ctrl Pts',(12.7926629650567,1.95339909479374,-3.05216148420481E-5));
#12447=CARTESIAN_POINT('Ctrl Pts',(12.7828174539371,1.94283764251631,0.201563933751552));
#12448=CARTESIAN_POINT('Ctrl Pts',(12.7729721028855,1.93227621586597,0.403158398304112));
#12449=CARTESIAN_POINT('Ctrl Pts',(12.7631269141765,1.92171481533599,0.604752872180064));
#12450=CARTESIAN_POINT('Ctrl Pts',(12.8889963716306,1.96391015057091,-1.66533453693773E-16));
#12451=CARTESIAN_POINT('Ctrl Pts',(12.878997439685,1.95334878321468,0.201594505478638));
#12452=CARTESIAN_POINT('Ctrl Pts',(12.8689986695886,1.94278744208894,0.403189020387166));
#12453=CARTESIAN_POINT('Ctrl Pts',(12.8590000636404,1.93222612769835,0.604783544866446));
#12454=CARTESIAN_POINT('',(12.8572578715866,1.93204080633595,0.60466226999893));
#12455=CARTESIAN_POINT('Ctrl Pts',(12.8889963716306,1.96391015057091,-3.88144377749811E-17));
#12456=CARTESIAN_POINT('Ctrl Pts',(12.8784169445746,1.95328733374019,0.201554108835021));
#12457=CARTESIAN_POINT('Ctrl Pts',(12.867837444884,1.94266422047353,0.403108198925375));
#12458=CARTESIAN_POINT('Ctrl Pts',(12.8572578715866,1.93204080633595,0.604662269998929));
#12459=CARTESIAN_POINT('Ctrl Pts',(12.8572578715866,1.93204080633595,0.60466226999893));
#12460=CARTESIAN_POINT('Ctrl Pts',(12.7715225733429,1.92264108900731,0.604675979983877));
#12461=CARTESIAN_POINT('Ctrl Pts',(12.6857696261193,1.91338852735451,0.604689390578107));
#12462=CARTESIAN_POINT('Ctrl Pts',(12.6000000000242,1.90428042250026,0.604702508168697));
#12463=CARTESIAN_POINT('Origin',(8.7,1.68851851851852,0.));
#12464=CARTESIAN_POINT('',(8.7,-1.5805153611151,0.605119933308333));
#12465=CARTESIAN_POINT('Ctrl Pts',(8.7,-1.5805153611151,0.605119933308333));
#12466=CARTESIAN_POINT('Ctrl Pts',(8.7,-1.58569938832865,0.504197823486131));
#12467=CARTESIAN_POINT('Ctrl Pts',(8.7,-1.59088373519313,0.403275164205241));
#12468=CARTESIAN_POINT('Ctrl Pts',(8.7,-1.60124586355191,0.201568897935389));
#12469=CARTESIAN_POINT('Ctrl Pts',(8.7,-1.60642370224807,0.10078416210737));
#12470=CARTESIAN_POINT('Ctrl Pts',(8.7,-1.61160179736194,0.));
#12471=CARTESIAN_POINT('',(8.7,-1.48045180431786,0.7));
#12472=CARTESIAN_POINT('Ctrl Pts',(8.70000000036779,-1.48045180452391,0.7));
#12473=CARTESIAN_POINT('Ctrl Pts',(8.70000000202598,-1.48836706478042,0.699999999180279));
#12474=CARTESIAN_POINT('Ctrl Pts',(8.70000127066624,-1.49622113223642,0.699007614827928));
#12475=CARTESIAN_POINT('Ctrl Pts',(8.70000237141531,-1.50387364922569,0.697121884028934));
#12476=CARTESIAN_POINT('Ctrl Pts',(8.70000291188189,-1.50763102664002,0.696195992283305));
#12477=CARTESIAN_POINT('Ctrl Pts',(8.70000341240591,-1.51133980954515,0.695053883793301));
#12478=CARTESIAN_POINT('Ctrl Pts',(8.70000377175886,-1.51498230649063,0.693702880475192));
#12479=CARTESIAN_POINT('Ctrl Pts',(8.70000450976793,-1.52246296255016,0.690928302676144));
#12480=CARTESIAN_POINT('Ctrl Pts',(8.70000452394134,-1.52958344744078,0.687306123577328));
#12481=CARTESIAN_POINT('Ctrl Pts',(8.70000379461986,-1.53619834892264,0.682919715776694));
#12482=CARTESIAN_POINT('Ctrl Pts',(8.70000333219987,-1.54039247012311,0.680138551763745));
#12483=CARTESIAN_POINT('Ctrl Pts',(8.70000258238552,-1.54438316197938,0.67704909562189));
#12484=CARTESIAN_POINT('Ctrl Pts',(8.70000192913237,-1.54812716280968,0.67366362845569));
#12485=CARTESIAN_POINT('Ctrl Pts',(8.70000138361353,-1.55125370412533,0.670836491537814));
#12486=CARTESIAN_POINT('Ctrl Pts',(8.70000090341281,-1.55418891097064,0.66782012731024));
#12487=CARTESIAN_POINT('Ctrl Pts',(8.7000009033621,-1.55691103280728,0.664625500020687));
#12488=CARTESIAN_POINT('Ctrl Pts',(8.7000009032669,-1.56202159382457,0.658627848677152));
#12489=CARTESIAN_POINT('Ctrl Pts',(8.70000241148087,-1.56638404855443,0.652003279246098));
#12490=CARTESIAN_POINT('Ctrl Pts',(8.70000292788623,-1.5699383402149,0.64491699469699));
#12491=CARTESIAN_POINT('Ctrl Pts',(8.70000298354275,-1.57032141040405,0.644153257609021));
#12492=CARTESIAN_POINT('Ctrl Pts',(8.70000303046442,-1.57069504840788,0.643384135640712));
#12493=CARTESIAN_POINT('Ctrl Pts',(8.70000306761332,-1.57105914547653,0.642609822781892));
#12494=CARTESIAN_POINT('Ctrl Pts',(8.70000341208914,-1.57443535963509,0.635429742901602));
#12495=CARTESIAN_POINT('Ctrl Pts',(8.70000263566904,-1.57695592401075,0.627888404173009));
#12496=CARTESIAN_POINT('Ctrl Pts',(8.70000151703179,-1.57856725066757,0.620153930269154));
#12497=CARTESIAN_POINT('Ctrl Pts',(8.70000080174396,-1.57959757782623,0.615208292159515));
#12498=CARTESIAN_POINT('Ctrl Pts',(8.7,-1.58025528705454,0.610183028431161));
#12499=CARTESIAN_POINT('Ctrl Pts',(8.7,-1.5805153611151,0.605119933308333));
#12500=CARTESIAN_POINT('',(8.7,1.48045180431904,0.7));
#12501=CARTESIAN_POINT('',(8.7,0.844259259259259,0.7));
#12502=CARTESIAN_POINT('',(8.7,1.5805153611151,0.605119933308333));
#12503=CARTESIAN_POINT('Ctrl Pts',(8.7,1.5805153611151,0.605119933308333));
#12504=CARTESIAN_POINT('Ctrl Pts',(8.7,1.58010890623597,0.61303275518587));
#12505=CARTESIAN_POINT('Ctrl Pts',(8.70000179355525,1.57873376841273,0.620855553142259));
#12506=CARTESIAN_POINT('Ctrl Pts',(8.7000025961206,1.5764741717406,0.62842799710221));
#12507=CARTESIAN_POINT('Ctrl Pts',(8.70000304562639,1.57520860278123,0.632669218617747));
#12508=CARTESIAN_POINT('Ctrl Pts',(8.70000324668712,1.57366457852079,0.636831947144834));
#12509=CARTESIAN_POINT('Ctrl Pts',(8.70000313318341,1.57185009366145,0.640886032861668));
#12510=CARTESIAN_POINT('Ctrl Pts',(8.70000293045856,1.56860930815545,0.648126888117959));
#12511=CARTESIAN_POINT('Ctrl Pts',(8.70000158438082,1.56454425420738,0.654942317779106));
#12512=CARTESIAN_POINT('Ctrl Pts',(8.70000106269264,1.55971945710293,0.661169479919421));
#12513=CARTESIAN_POINT('Ctrl Pts',(8.70000096439252,1.55881033523018,0.662342845179011));
#12514=CARTESIAN_POINT('Ctrl Pts',(8.70000090351839,1.55787410801649,0.663495254390581));
#12515=CARTESIAN_POINT('Ctrl Pts',(8.70000090409683,1.55691103285321,0.664625500020665));
#12516=CARTESIAN_POINT('Ctrl Pts',(8.70000090523835,1.55501044337284,0.666855993586132));
#12517=CARTESIAN_POINT('Ctrl Pts',(8.70000114361209,1.55300532702719,0.669000219206223));
#12518=CARTESIAN_POINT('Ctrl Pts',(8.70000146777886,1.55090303951829,0.671054438207787));
#12519=CARTESIAN_POINT('Ctrl Pts',(8.70000234447876,1.54521746205001,0.676610015749294));
#12520=CARTESIAN_POINT('Ctrl Pts',(8.70000370702799,1.53888821826629,0.681447385411957));
#12521=CARTESIAN_POINT('Ctrl Pts',(8.70000415375638,1.53207947242364,0.685512859850771));
#12522=CARTESIAN_POINT('Ctrl Pts',(8.70000443876751,1.52773551673798,0.688106618115728));
#12523=CARTESIAN_POINT('Ctrl Pts',(8.70000441165582,1.52319541573235,0.690385508075002));
#12524=CARTESIAN_POINT('Ctrl Pts',(8.70000407315693,1.51849599021366,0.692326230693156));
#12525=CARTESIAN_POINT('Ctrl Pts',(8.70000354533424,1.51116815716702,0.695352407250086));
#12526=CARTESIAN_POINT('Ctrl Pts',(8.70000225790696,1.50353761203248,0.697524030080351));
#12527=CARTESIAN_POINT('Ctrl Pts',(8.70000121423997,1.49575164755759,0.698771658000832));
#12528=CARTESIAN_POINT('Ctrl Pts',(8.70000053774506,1.49070486028667,0.699580358416591));
#12529=CARTESIAN_POINT('Ctrl Pts',(8.70000000144466,1.48559217323052,0.699999999467653));
#12530=CARTESIAN_POINT('Ctrl Pts',(8.70000000036779,1.48045180452391,0.7));
#12531=CARTESIAN_POINT('Ctrl Pts',(8.7,1.61160179736194,0.));
#12532=CARTESIAN_POINT('Ctrl Pts',(8.7,1.60642368739695,0.100784451162898));
#12533=CARTESIAN_POINT('Ctrl Pts',(8.7,1.60124583384883,0.201569476094892));
#12534=CARTESIAN_POINT('Ctrl Pts',(8.7,1.59088370548997,0.403275742430776));
#12535=CARTESIAN_POINT('Ctrl Pts',(8.7,1.58569937347746,0.504198112607714));
#12536=CARTESIAN_POINT('Ctrl Pts',(8.7,1.5805153611151,0.605119933308333));
#12537=CARTESIAN_POINT('Ctrl Pts',(8.7100201910492,-1.61222456240079,1.33887903992595E-6));
#12538=CARTESIAN_POINT('Ctrl Pts',(8.70667727354472,-1.60164608969543,0.201874135619687));
#12539=CARTESIAN_POINT('Ctrl Pts',(8.70333445073708,-1.59106762573893,0.40374693439627));
#12540=CARTESIAN_POINT('Ctrl Pts',(8.69999172399519,-1.58048917070122,0.605619735240497));
#12541=CARTESIAN_POINT('Ctrl Pts',(7.30266630830786,-1.52469223633113,-0.000186944012493601));
#12542=CARTESIAN_POINT('Ctrl Pts',(7.3015714609838,-1.51411327886182,0.201685539385837));
#12543=CARTESIAN_POINT('Ctrl Pts',(7.30047669312962,-1.50353432123569,0.403558023359813));
#12544=CARTESIAN_POINT('Ctrl Pts',(7.2993819983171,-1.49295537435081,0.605430507723141));
#12545=CARTESIAN_POINT('Ctrl Pts',(5.89591889571946,-1.46411055243784,-0.000276130330627546));
#12546=CARTESIAN_POINT('Ctrl Pts',(5.8970730573458,-1.45353136553189,0.201596203763285));
#12547=CARTESIAN_POINT('Ctrl Pts',(5.89822728315403,-1.44295217665945,0.403468537584815));
#12548=CARTESIAN_POINT('Ctrl Pts',(5.89938156763751,-1.43237299696387,0.60534087113472));
#12549=CARTESIAN_POINT('Ctrl Pts',(4.48978738186403,-1.41740792524342,-0.000330195618103912));
#12550=CARTESIAN_POINT('Ctrl Pts',(4.49319153668887,-1.4068286019831,0.201542048187911));
#12551=CARTESIAN_POINT('Ctrl Pts',(4.49659574248722,-1.39624928130228,0.403414291272231));
#12552=CARTESIAN_POINT('Ctrl Pts',(4.5,-1.3856699632509,0.605286533625018));
#12553=CARTESIAN_POINT('Ctrl Pts',(4.50000000014037,-1.38566996330298,0.605286533623957));
#12554=CARTESIAN_POINT('Ctrl Pts',(5.90109530155974,-1.43243455365708,0.605259331490037));
#12555=CARTESIAN_POINT('Ctrl Pts',(7.30150776148394,-1.49309969195427,0.605214402664297));
#12556=CARTESIAN_POINT('Ctrl Pts',(8.7,-1.5805153611151,0.605119933308333));
#12557=CARTESIAN_POINT('Ctrl Pts',(8.7062300060629,-1.48084102486261,0.7));
#12558=CARTESIAN_POINT('Ctrl Pts',(7.30535837857749,-1.39328148786737,0.7));
#12559=CARTESIAN_POINT('Ctrl Pts',(5.90286553803659,-1.3325543763676,0.7));
#12560=CARTESIAN_POINT('Ctrl Pts',(4.5,-1.28575421950843,0.7));
#12561=CARTESIAN_POINT('Ctrl Pts',(8.7044244076592,-1.50972892972339,0.7));
#12562=CARTESIAN_POINT('Ctrl Pts',(7.30392377861185,-1.42217417124324,0.699999322371676));
#12563=CARTESIAN_POINT('Ctrl Pts',(5.90170976758769,-1.36144968116949,0.700000194339816));
#12564=CARTESIAN_POINT('Ctrl Pts',(4.49903600403804,-1.314650633636,0.7));
#12565=CARTESIAN_POINT('Ctrl Pts',(8.70129509098077,-1.55979510296572,0.676577193851887));
#12566=CARTESIAN_POINT('Ctrl Pts',(7.30143307762773,-1.47225060169427,0.676608218952397));
#12567=CARTESIAN_POINT('Ctrl Pts',(5.89970879741633,-1.41153023905743,0.676622651488038));
#12568=CARTESIAN_POINT('Ctrl Pts',(4.49736521340071,-1.36473368385825,0.676631564755462));
#12569=CARTESIAN_POINT('Ctrl Pts',(8.70006933407556,-1.57940608001781,0.626799670546273));
#12570=CARTESIAN_POINT('Ctrl Pts',(7.3004573192207,-1.49190036240803,0.626879818917698));
#12571=CARTESIAN_POINT('Ctrl Pts',(5.89892183391985,-1.43119871194172,0.62691759730524));
#12572=CARTESIAN_POINT('Ctrl Pts',(4.49670869913724,-1.38441313147668,0.626940642142451));
#12573=CARTESIAN_POINT('Ctrl Pts',(8.7,-1.5805153611151,0.605119933308333));
#12574=CARTESIAN_POINT('Ctrl Pts',(7.30039998287682,-1.49303044794594,0.605214477495697));
#12575=CARTESIAN_POINT('Ctrl Pts',(5.89887670103551,-1.4323384618751,0.605259402637312));
#12576=CARTESIAN_POINT('Ctrl Pts',(4.49667047719213,-1.38555885946567,0.605286598232956));
#12577=CARTESIAN_POINT('Ctrl Pts',(8.70000000036771,-1.48045180452391,0.7));
#12578=CARTESIAN_POINT('Ctrl Pts',(7.30120024114866,-1.39310147361351,0.7));
#12579=CARTESIAN_POINT('Ctrl Pts',(5.90078591724148,-1.332484999384,0.7));
#12580=CARTESIAN_POINT('Ctrl Pts',(4.5,-1.28575421950843,0.7));
#12581=CARTESIAN_POINT('Origin',(6.87409734069396,-2.22251806091942E-16,
0.7));
#12582=CARTESIAN_POINT('Ctrl Pts',(4.5,1.28575421950843,0.7));
#12583=CARTESIAN_POINT('Ctrl Pts',(5.9007859172415,1.332484999384,0.7));
#12584=CARTESIAN_POINT('Ctrl Pts',(7.30120024114871,1.39310147361351,0.7));
#12585=CARTESIAN_POINT('Ctrl Pts',(8.70000000036779,1.48045180452391,0.7));
#12586=CARTESIAN_POINT('Ctrl Pts',(4.5,1.28575421950843,0.7));
#12587=CARTESIAN_POINT('Ctrl Pts',(5.90286553803659,1.3325543763676,0.7));
#12588=CARTESIAN_POINT('Ctrl Pts',(7.30535837857749,1.39328148786737,0.7));
#12589=CARTESIAN_POINT('Ctrl Pts',(8.7062300060629,1.48084102486261,0.7));
#12590=CARTESIAN_POINT('Ctrl Pts',(4.49903600403804,1.314650633636,0.7));
#12591=CARTESIAN_POINT('Ctrl Pts',(5.90170976758769,1.36144968116949,0.700000194339816));
#12592=CARTESIAN_POINT('Ctrl Pts',(7.30392377861185,1.42217417124324,0.699999322371676));
#12593=CARTESIAN_POINT('Ctrl Pts',(8.7044244076592,1.50972892972339,0.7));
#12594=CARTESIAN_POINT('Ctrl Pts',(4.49736521340071,1.36473368385825,0.676631564755462));
#12595=CARTESIAN_POINT('Ctrl Pts',(5.89970879741633,1.41153023905743,0.676622651488038));
#12596=CARTESIAN_POINT('Ctrl Pts',(7.30143307762774,1.47225060169427,0.676608218952397));
#12597=CARTESIAN_POINT('Ctrl Pts',(8.70129509098078,1.55979510296572,0.676577193851887));
#12598=CARTESIAN_POINT('Ctrl Pts',(4.49670869913724,1.38441313147668,0.626940642142451));
#12599=CARTESIAN_POINT('Ctrl Pts',(5.89892183391985,1.43119871194172,0.626917597305239));
#12600=CARTESIAN_POINT('Ctrl Pts',(7.3004573192207,1.49190036240803,0.626879818917698));
#12601=CARTESIAN_POINT('Ctrl Pts',(8.70006933407556,1.57940608001781,0.626799670546273));
#12602=CARTESIAN_POINT('Ctrl Pts',(4.49667047719213,1.38555885946567,0.605286598232956));
#12603=CARTESIAN_POINT('Ctrl Pts',(5.89887670103551,1.4323384618751,0.605259402637312));
#12604=CARTESIAN_POINT('Ctrl Pts',(7.30039998287682,1.49303044794594,0.605214477495697));
#12605=CARTESIAN_POINT('Ctrl Pts',(8.7,1.5805153611151,0.605119933308333));
#12606=CARTESIAN_POINT('Ctrl Pts',(8.7,1.5805153611151,0.605119933308333));
#12607=CARTESIAN_POINT('Ctrl Pts',(7.30150776148394,1.49309969195427,0.605214402664297));
#12608=CARTESIAN_POINT('Ctrl Pts',(5.90109530155974,1.43243455365708,0.605259331490037));
#12609=CARTESIAN_POINT('Ctrl Pts',(4.50000000014037,1.38566996330298,0.605286533623957));
#12610=CARTESIAN_POINT('Ctrl Pts',(4.48978738186405,1.41740792524342,-0.00033019561810394));
#12611=CARTESIAN_POINT('Ctrl Pts',(4.49319153668889,1.40682860198312,0.201542048187577));
#12612=CARTESIAN_POINT('Ctrl Pts',(4.49659574248723,1.39624928130232,0.403414291271564));
#12613=CARTESIAN_POINT('Ctrl Pts',(4.5,1.38566996325095,0.605286533624017));
#12614=CARTESIAN_POINT('Ctrl Pts',(5.89591889571947,1.46411055243784,-0.000276130330627574));
#12615=CARTESIAN_POINT('Ctrl Pts',(5.89707305734581,1.45353136553191,0.201596203762952));
#12616=CARTESIAN_POINT('Ctrl Pts',(5.89822728315404,1.44295217665948,0.403468537584147));
#12617=CARTESIAN_POINT('Ctrl Pts',(5.89938156763751,1.43237299696393,0.605340871133719));
#12618=CARTESIAN_POINT('Ctrl Pts',(7.30266630830786,1.52469223633113,-0.000186944012493549));
#12619=CARTESIAN_POINT('Ctrl Pts',(7.3015714609838,1.51411327886184,0.201685539385503));
#12620=CARTESIAN_POINT('Ctrl Pts',(7.30047669312963,1.50353432123572,0.403558023359145));
#12621=CARTESIAN_POINT('Ctrl Pts',(7.29938199831711,1.49295537435086,0.60543050772214));
#12622=CARTESIAN_POINT('Ctrl Pts',(8.7100201910492,1.61222456240079,1.33887903989646E-6));
#12623=CARTESIAN_POINT('Ctrl Pts',(8.70667727354472,1.60164608969545,0.201874135619353));
#12624=CARTESIAN_POINT('Ctrl Pts',(8.7033344507371,1.59106762573896,0.403746934395602));
#12625=CARTESIAN_POINT('Ctrl Pts',(8.6999917239952,1.58048917070127,0.605619735239495));
#12626=CARTESIAN_POINT('Origin',(4.3,1.48481481481482,0.));
#12627=CARTESIAN_POINT('',(4.3,-1.37908752581626,0.605290299758539));
#12628=CARTESIAN_POINT('Ctrl Pts',(4.3,-1.37908752581626,0.605290299758539));
#12629=CARTESIAN_POINT('Ctrl Pts',(4.3,-1.38444464017247,0.504222347694443));
#12630=CARTESIAN_POINT('Ctrl Pts',(4.3,-1.38980163214303,0.403154389143214));
#12631=CARTESIAN_POINT('Ctrl Pts',(4.3,-1.40049562949383,0.201390955816302));
#12632=CARTESIAN_POINT('Ctrl Pts',(4.3,-1.40583263576898,0.100695481088992));
#12633=CARTESIAN_POINT('Ctrl Pts',(4.3,-1.41116952203211,0.));
#12634=CARTESIAN_POINT('Ctrl Pts',(4.30000000005992,-1.27917501058303,0.7));
#12635=CARTESIAN_POINT('Ctrl Pts',(4.30000000048661,-1.28708628524264,0.699999999884766));
#12636=CARTESIAN_POINT('Ctrl Pts',(4.30000064978116,-1.29493415608545,0.69900616264686));
#12637=CARTESIAN_POINT('Ctrl Pts',(4.30000121018478,-1.30257825621016,0.697119208693397));
#12638=CARTESIAN_POINT('Ctrl Pts',(4.30000152558655,-1.30688044586137,0.696057208766858));
#12639=CARTESIAN_POINT('Ctrl Pts',(4.30000181105247,-1.31111814675806,0.694711271736901));
#12640=CARTESIAN_POINT('Ctrl Pts',(4.30000199036827,-1.31526464671957,0.693092387263961));
#12641=CARTESIAN_POINT('Ctrl Pts',(4.30000231141323,-1.32268849323592,0.690193954859197));
#12642=CARTESIAN_POINT('Ctrl Pts',(4.30000222777046,-1.32973966400828,0.686455190804221));
#12643=CARTESIAN_POINT('Ctrl Pts',(4.30000179417102,-1.33627196700415,0.681957645816867));
#12644=CARTESIAN_POINT('Ctrl Pts',(4.30000155535849,-1.33986974800182,0.679480543652151));
#12645=CARTESIAN_POINT('Ctrl Pts',(4.30000121902461,-1.34330986828215,0.67677238407294));
#12646=CARTESIAN_POINT('Ctrl Pts',(4.30000092191081,-1.34656397897095,0.673841242448196));
#12647=CARTESIAN_POINT('Ctrl Pts',(4.30000063243573,-1.34973442737118,0.670985459666446));
#12648=CARTESIAN_POINT('Ctrl Pts',(4.30000037658882,-1.35270906921767,0.667935271966333));
#12649=CARTESIAN_POINT('Ctrl Pts',(4.30000037869864,-1.35546536049262,0.66470214425512));
#12650=CARTESIAN_POINT('Ctrl Pts',(4.30000038260995,-1.36057515211559,0.658708362304413));
#12651=CARTESIAN_POINT('Ctrl Pts',(4.30000117797282,-1.36493744806469,0.652087250959406));
#12652=CARTESIAN_POINT('Ctrl Pts',(4.30000145944905,-1.36849285270534,0.645004510397983));
#12653=CARTESIAN_POINT('Ctrl Pts',(4.30000148826005,-1.36885677248754,0.644279543857467));
#12654=CARTESIAN_POINT('Ctrl Pts',(4.30000151299237,-1.36921219826683,0.643549721050429));
#12655=CARTESIAN_POINT('Ctrl Pts',(4.30000153317099,-1.36955903781249,0.642815208524159));
#12656=CARTESIAN_POINT('Ctrl Pts',(4.30000173031152,-1.37294758118467,0.635639188419686));
#12657=CARTESIAN_POINT('Ctrl Pts',(4.30000134819424,-1.37548140076902,0.628100134775109));
#12658=CARTESIAN_POINT('Ctrl Pts',(4.30000077902196,-1.37710733725971,0.620366659714886));
#12659=CARTESIAN_POINT('Ctrl Pts',(4.30000041405338,-1.37814993145247,0.615407747584041));
#12660=CARTESIAN_POINT('Ctrl Pts',(4.3,-1.37881837002099,0.610368224776708));
#12661=CARTESIAN_POINT('Ctrl Pts',(4.3,-1.37908752581626,0.605290299758539));
#12662=CARTESIAN_POINT('',(4.3,1.37908752581626,0.605290299758539));
#12663=CARTESIAN_POINT('Ctrl Pts',(4.3,1.37908752581626,0.605290299758539));
#12664=CARTESIAN_POINT('Ctrl Pts',(4.3,1.37866806817032,0.613203837240499));
#12665=CARTESIAN_POINT('Ctrl Pts',(4.30000092021544,1.37728139671899,0.621026590428679));
#12666=CARTESIAN_POINT('Ctrl Pts',(4.30000132151137,1.37501133257008,0.628597948954885));
#12667=CARTESIAN_POINT('Ctrl Pts',(4.30000154544343,1.37374458621782,0.632822935636113));
#12668=CARTESIAN_POINT('Ctrl Pts',(4.30000164013187,1.37220176226583,0.636969676056352));
#12669=CARTESIAN_POINT('Ctrl Pts',(4.30000157305315,1.37039070587839,0.641008268098125));
#12670=CARTESIAN_POINT('Ctrl Pts',(4.30000145288191,1.36714620633991,0.648243387946652));
#12671=CARTESIAN_POINT('Ctrl Pts',(4.30000073948134,1.36307905360626,0.655053358422861));
#12672=CARTESIAN_POINT('Ctrl Pts',(4.3000004635866,1.35825284513469,0.661274801567968));
#12673=CARTESIAN_POINT('Ctrl Pts',(4.30000041199046,1.35735027731582,0.662438297592388));
#12674=CARTESIAN_POINT('Ctrl Pts',(4.30000037986005,1.35642103364291,0.663581140343808));
#12675=CARTESIAN_POINT('Ctrl Pts',(4.30000037943224,1.35546536051643,0.664702144255114));
#12676=CARTESIAN_POINT('Ctrl Pts',(4.300000378582,1.3535659898678,0.666930104702213));
#12677=CARTESIAN_POINT('Ctrl Pts',(4.3000005018795,1.35156225525783,0.669071850305581));
#12678=CARTESIAN_POINT('Ctrl Pts',(4.30000067038034,1.34946148384904,0.671123623013939));
#12679=CARTESIAN_POINT('Ctrl Pts',(4.30000112630012,1.34377733881547,0.676675190215126));
#12680=CARTESIAN_POINT('Ctrl Pts',(4.30000183907902,1.33744971106208,0.68150833207295));
#12681=CARTESIAN_POINT('Ctrl Pts',(4.30000208123143,1.33064243458576,0.685568782013219));
#12682=CARTESIAN_POINT('Ctrl Pts',(4.30000223513396,1.3263159977886,0.688149444058562));
#12683=CARTESIAN_POINT('Ctrl Pts',(4.3000022300233,1.32179485563522,0.690417305529342));
#12684=CARTESIAN_POINT('Ctrl Pts',(4.30000206344016,1.31711540146937,0.692349146556373));
#12685=CARTESIAN_POINT('Ctrl Pts',(4.3000018029167,1.30979708846622,0.695370400063095));
#12686=CARTESIAN_POINT('Ctrl Pts',(4.30000114702936,1.30217656646843,0.69753735975804));
#12687=CARTESIAN_POINT('Ctrl Pts',(4.3000006156201,1.29440092269557,0.69878042986007));
#12688=CARTESIAN_POINT('Ctrl Pts',(4.30000027236218,1.28937833178082,0.699583377215073));
#12689=CARTESIAN_POINT('Ctrl Pts',(4.30000000033581,1.28429042584107,0.69999999992549));
#12690=CARTESIAN_POINT('Ctrl Pts',(4.30000000005992,1.27917501058303,0.7));
#12691=CARTESIAN_POINT('Ctrl Pts',(4.3,1.41116952203211,0.));
#12692=CARTESIAN_POINT('Ctrl Pts',(4.3,1.40583262613343,0.100695662891028));
#12693=CARTESIAN_POINT('Ctrl Pts',(4.3,1.40049561022223,0.201391319421434));
#12694=CARTESIAN_POINT('Ctrl Pts',(4.3,1.38980161287056,0.403154752748307));
#12695=CARTESIAN_POINT('Ctrl Pts',(4.3,1.38444463053604,0.504222529496425));
#12696=CARTESIAN_POINT('Ctrl Pts',(4.3,1.37908752581626,0.605290299758539));
#12697=CARTESIAN_POINT('Ctrl Pts',(4.3,-1.41116952203217,-1.08233907947231E-12));
#12698=CARTESIAN_POINT('Ctrl Pts',(4.30370667985561,-1.40059355144761,0.201807922462111));
#12699=CARTESIAN_POINT('Ctrl Pts',(4.30741340932898,-1.39001758331341,0.403615844144917));
#12700=CARTESIAN_POINT('Ctrl Pts',(4.31112018914117,-1.37944161767694,0.605423765036612));
#12701=CARTESIAN_POINT('Ctrl Pts',(3.22410085073145,-1.37636920007795,-3.90459529712038E-5));
#12702=CARTESIAN_POINT('Ctrl Pts',(3.2295286994181,-1.36579313421488,0.201768811380596));
#12703=CARTESIAN_POINT('Ctrl Pts',(3.23495659078338,-1.35521706809947,0.403576667516588));
#12704=CARTESIAN_POINT('Ctrl Pts',(3.24038452463065,-1.34464100578453,0.605384522622892));
#12705=CARTESIAN_POINT('Ctrl Pts',(2.14856196511704,-1.34935185539723,-5.92140864038068E-5));
#12706=CARTESIAN_POINT('Ctrl Pts',(2.15571155670467,-1.33877574824886,0.201748609775608));
#12707=CARTESIAN_POINT('Ctrl Pts',(2.16286118630165,-1.32819964054015,0.403556432267456));
#12708=CARTESIAN_POINT('Ctrl Pts',(2.17001085376486,-1.31762353633116,0.605364253566666));
#12709=CARTESIAN_POINT('Ctrl Pts',(1.073384157387,-1.32427529283232,-8.86713468529234E-5));
#12710=CARTESIAN_POINT('Ctrl Pts',(1.08225606990756,-1.31369916974321,0.201719104822629));
#12711=CARTESIAN_POINT('Ctrl Pts',(1.09112801825726,-1.30312304798914,0.403526879488275));
#12712=CARTESIAN_POINT('Ctrl Pts',(1.10000000295732,-1.29254692759565,0.605334652628532));
#12713=CARTESIAN_POINT('Ctrl Pts',(1.10000000298281,-1.29254692760111,0.605334652628557));
#12714=CARTESIAN_POINT('Ctrl Pts',(2.16694388170712,-1.31755402957363,0.605319894542965));
#12715=CARTESIAN_POINT('Ctrl Pts',(3.23367147240841,-1.34448060345116,0.605309774863278));
#12716=CARTESIAN_POINT('Ctrl Pts',(4.3,-1.37908752581626,0.605290299758539));
#12717=CARTESIAN_POINT('Ctrl Pts',(4.30323908112369,-1.2792801058419,0.7));
#12718=CARTESIAN_POINT('Ctrl Pts',(3.23565147654712,-1.24463335454069,0.7));
#12719=CARTESIAN_POINT('Ctrl Pts',(2.1678436779024,-1.21768649131741,0.7));
#12720=CARTESIAN_POINT('Ctrl Pts',(1.09999999999999,-1.19266190204553,0.7));
#12721=CARTESIAN_POINT('Ctrl Pts',(4.30230129178181,-1.30817667592415,0.7));
#12722=CARTESIAN_POINT('Ctrl Pts',(3.23485320804887,-1.27353066282864,0.699999860738333));
#12723=CARTESIAN_POINT('Ctrl Pts',(2.16713169816659,-1.24658393122273,0.700000105496227));
#12724=CARTESIAN_POINT('Ctrl Pts',(1.0993228455422,-1.22155728565617,0.7));
#12725=CARTESIAN_POINT('Ctrl Pts',(4.30067574076257,-1.35826558912881,0.676637683834297));
#12726=CARTESIAN_POINT('Ctrl Pts',(3.23346787205668,-1.32362126434549,0.676644071225102));
#12727=CARTESIAN_POINT('Ctrl Pts',(2.16589795861771,-1.29667457247055,0.676647306834711));
#12728=CARTESIAN_POINT('Ctrl Pts',(1.09814906228501,-1.27164470234869,0.676652147774997));
#12729=CARTESIAN_POINT('Ctrl Pts',(4.30003720890047,-1.37794098943329,0.626943772371838));
#12730=CARTESIAN_POINT('Ctrl Pts',(3.23292426239396,-1.34330449078822,0.626960286972675));
#12731=CARTESIAN_POINT('Ctrl Pts',(2.16541285690349,-1.31636171257899,0.6269687859393));
#12732=CARTESIAN_POINT('Ctrl Pts',(1.09768760301306,-1.29133598921902,0.626981304916489));
#12733=CARTESIAN_POINT('Ctrl Pts',(4.3,-1.37908752581626,0.605290299758539));
#12734=CARTESIAN_POINT('Ctrl Pts',(3.23289209128077,-1.34445530919946,0.605309789097661));
#12735=CARTESIAN_POINT('Ctrl Pts',(2.16538453588699,-1.31751467232976,0.605319909330946));
#12736=CARTESIAN_POINT('Ctrl Pts',(1.09766050997011,-1.29249209748956,0.605334684996117));
#12737=CARTESIAN_POINT('Ctrl Pts',(1.09999999999999,1.19266190204553,0.7));
#12738=CARTESIAN_POINT('Ctrl Pts',(2.1678436779024,1.21768649131741,0.7));
#12739=CARTESIAN_POINT('Ctrl Pts',(3.23565147654712,1.24463335454069,0.7));
#12740=CARTESIAN_POINT('Ctrl Pts',(4.30323908112369,1.2792801058419,0.7));
#12741=CARTESIAN_POINT('Ctrl Pts',(1.0993228455422,1.22155728565617,0.7));
#12742=CARTESIAN_POINT('Ctrl Pts',(2.16713169816659,1.24658393122273,0.700000105496227));
#12743=CARTESIAN_POINT('Ctrl Pts',(3.23485320804887,1.27353066282864,0.699999860738333));
#12744=CARTESIAN_POINT('Ctrl Pts',(4.30230129178181,1.30817667592415,0.7));
#12745=CARTESIAN_POINT('Ctrl Pts',(1.09814906228501,1.27164470234869,0.676652147774997));
#12746=CARTESIAN_POINT('Ctrl Pts',(2.16589795861771,1.29667457247055,0.676647306834711));
#12747=CARTESIAN_POINT('Ctrl Pts',(3.23346787205668,1.32362126434549,0.676644071225102));
#12748=CARTESIAN_POINT('Ctrl Pts',(4.30067574076257,1.35826558912881,0.676637683834297));
#12749=CARTESIAN_POINT('Ctrl Pts',(1.09768760301306,1.29133598921902,0.626981304916489));
#12750=CARTESIAN_POINT('Ctrl Pts',(2.16541285690349,1.31636171257899,0.6269687859393));
#12751=CARTESIAN_POINT('Ctrl Pts',(3.23292426239396,1.34330449078822,0.626960286972675));
#12752=CARTESIAN_POINT('Ctrl Pts',(4.30003720890047,1.37794098943329,0.626943772371838));
#12753=CARTESIAN_POINT('Ctrl Pts',(1.09766050997011,1.29249209748956,0.605334684996117));
#12754=CARTESIAN_POINT('Ctrl Pts',(2.16538453588699,1.31751467232976,0.605319909330946));
#12755=CARTESIAN_POINT('Ctrl Pts',(3.23289209128077,1.34445530919946,0.605309789097661));
#12756=CARTESIAN_POINT('Ctrl Pts',(4.3,1.37908752581626,0.605290299758539));
#12757=CARTESIAN_POINT('Ctrl Pts',(4.3,1.37908752581626,0.605290299758539));
#12758=CARTESIAN_POINT('Ctrl Pts',(3.23367147240841,1.34448060345116,0.605309774863278));
#12759=CARTESIAN_POINT('Ctrl Pts',(2.16694388170711,1.31755402957363,0.605319894542965));
#12760=CARTESIAN_POINT('Ctrl Pts',(1.10000000298281,1.29254692760111,0.605334652628557));
#12761=CARTESIAN_POINT('Ctrl Pts',(1.07338415738705,1.32427529283227,-8.86713457716078E-5));
#12762=CARTESIAN_POINT('Ctrl Pts',(1.08225606990759,1.31369916974318,0.201719104823349));
#12763=CARTESIAN_POINT('Ctrl Pts',(1.09112801825728,1.30312304798912,0.403526879488635));
#12764=CARTESIAN_POINT('Ctrl Pts',(1.10000000295732,1.29254692759565,0.605334652628532));
#12765=CARTESIAN_POINT('Ctrl Pts',(2.14856196511707,1.34935185539717,-5.92140853224782E-5));
#12766=CARTESIAN_POINT('Ctrl Pts',(2.15571155670469,1.33877574824882,0.201748609776328));
#12767=CARTESIAN_POINT('Ctrl Pts',(2.16286118630166,1.32819964054013,0.403556432267816));
#12768=CARTESIAN_POINT('Ctrl Pts',(2.17001085376486,1.31762353633116,0.605364253566666));
#12769=CARTESIAN_POINT('Ctrl Pts',(3.22410085073147,1.37636920007789,-3.90459518899617E-5));
#12770=CARTESIAN_POINT('Ctrl Pts',(3.22952869941811,1.36579313421484,0.201768811381317));
#12771=CARTESIAN_POINT('Ctrl Pts',(3.23495659078338,1.35521706809945,0.403576667516948));
#12772=CARTESIAN_POINT('Ctrl Pts',(3.24038452463064,1.34464100578453,0.605384522622892));
#12773=CARTESIAN_POINT('Ctrl Pts',(4.3,1.41116952203211,-1.07899800205757E-15));
#12774=CARTESIAN_POINT('Ctrl Pts',(4.3037066798556,1.40059355144758,0.201807922462832));
#12775=CARTESIAN_POINT('Ctrl Pts',(4.30741340932897,1.39001758331339,0.403615844145277));
#12776=CARTESIAN_POINT('Ctrl Pts',(4.31112018914115,1.37944161767694,0.605423765036611));
#12777=CARTESIAN_POINT('Origin',(0.9,1.39290118819044,0.));
#12778=CARTESIAN_POINT('',(0.900000001878204,-1.28788040994396,0.605337476551879));
#12779=CARTESIAN_POINT('Ctrl Pts',(0.900000001878204,-1.28788040994396,
0.605337476551879));
#12780=CARTESIAN_POINT('Ctrl Pts',(0.900000001878204,-1.29328625806092,
0.504228160928694));
#12781=CARTESIAN_POINT('Ctrl Pts',(0.899999999999999,-1.29869191435855,
0.403118132397745));
#12782=CARTESIAN_POINT('Ctrl Pts',(0.899999999999999,-1.30947917558554,
0.201339438823693));
#12783=CARTESIAN_POINT('Ctrl Pts',(0.9,-1.31486085669789,0.100669384150719));
#12784=CARTESIAN_POINT('Ctrl Pts',(0.9,-1.32024227787037,0.));
#12785=CARTESIAN_POINT('',(0.9,-1.18799600975353,0.7));
#12786=CARTESIAN_POINT('Ctrl Pts',(0.900000000000324,-1.18799600975363,
0.7));
#12787=CARTESIAN_POINT('Ctrl Pts',(0.900000000063601,-1.19590581948314,
0.699999999935493));
#12788=CARTESIAN_POINT('Ctrl Pts',(0.900000451671414,-1.20375274583281,
0.699006541951706));
#12789=CARTESIAN_POINT('Ctrl Pts',(0.900000834722547,-1.21139610511184,
0.697120084132161));
#12790=CARTESIAN_POINT('Ctrl Pts',(0.900001049758257,-1.21568690349652,
0.696061072005504));
#12791=CARTESIAN_POINT('Ctrl Pts',(0.900001241882928,-1.21991360580594,
0.694719604949841));
#12792=CARTESIAN_POINT('Ctrl Pts',(0.900001357948449,-1.22404965357203,
0.693106547509926));
#12793=CARTESIAN_POINT('Ctrl Pts',(0.900001566283472,-1.23147376710855,
0.690211145364658));
#12794=CARTESIAN_POINT('Ctrl Pts',(0.900001483882417,-1.23852542365708,
0.686475281350474));
#12795=CARTESIAN_POINT('Ctrl Pts',(0.90000115772027,-1.24505817055452,0.681980323292531));
#12796=CARTESIAN_POINT('Ctrl Pts',(0.90000097852015,-1.2486473946309,0.67951070187031));
#12797=CARTESIAN_POINT('Ctrl Pts',(0.900000731874511,-1.25207971535834,
0.676811055842604));
#12798=CARTESIAN_POINT('Ctrl Pts',(0.90000051586667,-1.25532695882913,0.673889369778116));
#12799=CARTESIAN_POINT('Ctrl Pts',(0.900000304282776,-1.25850769714062,
0.671027521295527));
#12800=CARTESIAN_POINT('Ctrl Pts',(0.900000119565725,-1.26149151526032,
0.667969976014938));
#12801=CARTESIAN_POINT('Ctrl Pts',(0.900000124706954,-1.26425564062679,
0.664728268702146));
#12802=CARTESIAN_POINT('Ctrl Pts',(0.900000134210909,-1.26936533657602,
0.658735726205464));
#12803=CARTESIAN_POINT('Ctrl Pts',(0.900000724431276,-1.2737272220214,0.652115259198653));
#12804=CARTESIAN_POINT('Ctrl Pts',(0.900000949945503,-1.27728244659665,
0.645033014705304));
#12805=CARTESIAN_POINT('Ctrl Pts',(0.900000972753073,-1.27764200720725,
0.644316745985709));
#12806=CARTESIAN_POINT('Ctrl Pts',(0.900000992743332,-1.27799327761064,
0.64359573459864));
#12807=CARTESIAN_POINT('Ctrl Pts',(0.900001009576454,-1.27833616945273,
0.642870141642621));
#12808=CARTESIAN_POINT('Ctrl Pts',(0.900001176059944,-1.28172744954266,
0.635693858502874));
#12809=CARTESIAN_POINT('Ctrl Pts',(0.900000930108723,-1.28426399347052,
0.628153947608977));
#12810=CARTESIAN_POINT('Ctrl Pts',(0.900000539908504,-1.2858931319598,0.620419547606466));
#12811=CARTESIAN_POINT('Ctrl Pts',(0.900000289636433,-1.28693805157347,
0.615458750034127));
#12812=CARTESIAN_POINT('Ctrl Pts',(0.900000000000001,-1.28760881677759,
0.610417269724172));
#12813=CARTESIAN_POINT('Ctrl Pts',(0.900000000000001,-1.28788040985668,
0.605337476551933));
#12814=CARTESIAN_POINT('',(0.9,1.18799600975353,0.7));
#12815=CARTESIAN_POINT('',(0.9,0.696450594095222,0.7));
#12816=CARTESIAN_POINT('',(0.900000001878204,1.28788040994396,0.605337476551879));
#12817=CARTESIAN_POINT('Ctrl Pts',(0.900000000000001,1.28788040985668,0.605337476551933));
#12818=CARTESIAN_POINT('Ctrl Pts',(0.900000000000001,1.28745726486871,0.613251849878237));
#12819=CARTESIAN_POINT('Ctrl Pts',(0.900000641820462,1.28606767879774,0.621075732439556));
#12820=CARTESIAN_POINT('Ctrl Pts',(0.900000906166769,1.28379497466322,0.628648019961568));
#12821=CARTESIAN_POINT('Ctrl Pts',(0.900001053446495,1.2825287445946,0.632866896498568));
#12822=CARTESIAN_POINT('Ctrl Pts',(0.900001106693909,1.28098738700664,0.637007708770872));
#12823=CARTESIAN_POINT('Ctrl Pts',(0.900001044867119,1.27917862712792,0.641040603354488));
#12824=CARTESIAN_POINT('Ctrl Pts',(0.900000933962191,1.27593407274945,0.64827481168313));
#12825=CARTESIAN_POINT('Ctrl Pts',(0.900000399592996,1.27186725264719,0.655083885116145));
#12826=CARTESIAN_POINT('Ctrl Pts',(0.900000190596867,1.2670411556595,0.661303993035384));
#12827=CARTESIAN_POINT('Ctrl Pts',(0.900000151538061,1.26613921747962,0.662466454716044));
#12828=CARTESIAN_POINT('Ctrl Pts',(0.900000126821978,1.26521063179286,0.663608275427336));
#12829=CARTESIAN_POINT('Ctrl Pts',(0.900000125264574,1.26425564063975,0.664728268702142));
#12830=CARTESIAN_POINT('Ctrl Pts',(0.90000012217056,1.26235840892454,0.66695330163032));
#12831=CARTESIAN_POINT('Ctrl Pts',(0.900000209712012,1.26035699384613,0.66909223571964));
#12832=CARTESIAN_POINT('Ctrl Pts',(0.900000331194293,1.2582587086698,0.671141334714948));
#12833=CARTESIAN_POINT('Ctrl Pts',(0.900000660246931,1.25257519443757,0.676691620936499));
#12834=CARTESIAN_POINT('Ctrl Pts',(0.900001184896248,1.24624785575673,0.681523125886843));
#12835=CARTESIAN_POINT('Ctrl Pts',(0.900001377531805,1.23944073409582,0.685581770965975));
#12836=CARTESIAN_POINT('Ctrl Pts',(0.900001499905572,1.2351164383281,0.68816006802201));
#12837=CARTESIAN_POINT('Ctrl Pts',(0.900001510509735,1.23059756718463,0.690425789971136));
#12838=CARTESIAN_POINT('Ctrl Pts',(0.900001405318139,1.22592052877826,0.692355791713551));
#12839=CARTESIAN_POINT('Ctrl Pts',(0.900001240727996,1.21860250674997,0.695375607682216));
#12840=CARTESIAN_POINT('Ctrl Pts',(0.900000792095824,1.21098234272326,0.697541065921879));
#12841=CARTESIAN_POINT('Ctrl Pts',(0.900000425437202,1.20320741268883,0.698782789564668));
#12842=CARTESIAN_POINT('Ctrl Pts',(0.900000188792485,1.19818940410026,0.699584208982791));
#12843=CARTESIAN_POINT('Ctrl Pts',(0.900000000041206,1.19310633605572,0.699999999958324));
#12844=CARTESIAN_POINT('Ctrl Pts',(0.900000000000325,1.18799600975363,0.7));
#12845=CARTESIAN_POINT('Ctrl Pts',(0.9,1.32024227787037,0.));
#12846=CARTESIAN_POINT('Ctrl Pts',(0.9,1.31486080448354,0.100670360916234));
#12847=CARTESIAN_POINT('Ctrl Pts',(0.9,1.30947907114291,0.201341392534));
#12848=CARTESIAN_POINT('Ctrl Pts',(0.9,1.2986918099064,0.403120086121531));
#12849=CARTESIAN_POINT('Ctrl Pts',(0.900000001878204,1.29328620583358,0.504229137772713));
#12850=CARTESIAN_POINT('Ctrl Pts',(0.900000001878204,1.28788040994396,0.605337476551879));
#12851=CARTESIAN_POINT('Ctrl Pts',(0.899999999999997,-1.32024227787137,
-1.86669707469278E-11));
#12852=CARTESIAN_POINT('Ctrl Pts',(0.909148787559422,-1.30966717532842,
0.201788252636133));
#12853=CARTESIAN_POINT('Ctrl Pts',(0.91829761066914,-1.29909207410335,0.403576503749508));
#12854=CARTESIAN_POINT('Ctrl Pts',(0.92744646984625,-1.28851697422138,0.605364753299354));
#12855=CARTESIAN_POINT('Ctrl Pts',(0.699273108318574,-1.31559634352334,
-5.7001548815619E-6));
#12856=CARTESIAN_POINT('Ctrl Pts',(0.708743431409066,-1.30502123870946,
0.20178254329682));
#12857=CARTESIAN_POINT('Ctrl Pts',(0.718213789763005,-1.2944461351935,0.403570785162392));
#12858=CARTESIAN_POINT('Ctrl Pts',(0.727684183892774,-1.28387103300525,
0.605359025419352));
#12859=CARTESIAN_POINT('Ctrl Pts',(0.498558799217305,-1.31100715552056,
-1.1774619888836E-5));
#12860=CARTESIAN_POINT('Ctrl Pts',(0.508350677965937,-1.30043204942944,
0.201776459055217));
#12861=CARTESIAN_POINT('Ctrl Pts',(0.518142591787393,-1.28985694462582,
0.403564691096996));
#12862=CARTESIAN_POINT('Ctrl Pts',(0.527934541191295,-1.27928184113929,
0.60535292148228));
#12863=CARTESIAN_POINT('Ctrl Pts',(0.29785707328833,-1.3064367443434,-1.84041486642056E-5));
#12864=CARTESIAN_POINT('Ctrl Pts',(0.307970527825607,-1.29586163794,0.20176981888596));
#12865=CARTESIAN_POINT('Ctrl Pts',(0.318084017341356,-1.28528653282298,
0.403558040236175));
#12866=CARTESIAN_POINT('Ctrl Pts',(0.328197542344371,-1.27471142901691,
0.605346259877786));
#12867=CARTESIAN_POINT('',(0.32957180616905,-1.2747428754212,0.605346305703265));
#12868=CARTESIAN_POINT('Ctrl Pts',(0.297857995688647,-1.306435779838,1.57426155444895E-16));
#12869=CARTESIAN_POINT('Ctrl Pts',(0.308429283449307,-1.29587142805659,
0.201782098465301));
#12870=CARTESIAN_POINT('Ctrl Pts',(0.319000553694994,-1.28530712634462,
0.403564200350135));
#12871=CARTESIAN_POINT('Ctrl Pts',(0.329571806169048,-1.2747428754212,0.605346305703266));
#12872=CARTESIAN_POINT('Ctrl Pts',(0.32957180616905,-1.2747428754212,0.605346305703265));
#12873=CARTESIAN_POINT('Ctrl Pts',(0.519721397561595,-1.27909449722757,
0.60534313598158));
#12874=CARTESIAN_POINT('Ctrl Pts',(0.709864288600121,-1.28346276435313,
0.605340219076093));
#12875=CARTESIAN_POINT('Ctrl Pts',(0.900000001879218,-1.28788040990034,
0.605337476551906));
#12876=CARTESIAN_POINT('Ctrl Pts',(0.90231940407953,-1.18804989493878,0.7));
#12877=CARTESIAN_POINT('Ctrl Pts',(0.712166351817731,-1.18363199317816,
0.7));
#12878=CARTESIAN_POINT('Ctrl Pts',(0.522011847238247,-1.17926361631973,
0.7));
#12879=CARTESIAN_POINT('Ctrl Pts',(0.331856371369203,-1.17491202960101,
0.7));
#12880=CARTESIAN_POINT('Ctrl Pts',(0.901648075315333,-1.21694488185794,
0.7));
#12881=CARTESIAN_POINT('Ctrl Pts',(0.711500071980331,-1.21252656425213,
0.69999998041973));
#12882=CARTESIAN_POINT('Ctrl Pts',(0.521348914609444,-1.20815772874132,
0.700000022626678));
#12883=CARTESIAN_POINT('Ctrl Pts',(0.331195161244126,-1.20380556524924,
0.7));
#12884=CARTESIAN_POINT('Ctrl Pts',(0.900484091294294,-1.26704448261357,
0.676664431332699));
#12885=CARTESIAN_POINT('Ctrl Pts',(0.710344780071471,-1.26262550764723,
0.676665329845182));
#12886=CARTESIAN_POINT('Ctrl Pts',(0.520199507967113,-1.25825584722226,
0.676666267597974));
#12887=CARTESIAN_POINT('Ctrl Pts',(0.3300487189482,-1.25390275839508,0.676667306001616));
#12888=CARTESIAN_POINT('Ctrl Pts',(0.90002687589075,-1.28672371253673,0.626983665342106));
#12889=CARTESIAN_POINT('Ctrl Pts',(0.709890987426059,-1.28230548388611,
0.626985988983916));
#12890=CARTESIAN_POINT('Ctrl Pts',(0.519747959090447,-1.27793661492756,
0.626988445273931));
#12891=CARTESIAN_POINT('Ctrl Pts',(0.329598318905021,-1.27358432286302,
0.626991130804315));
#12892=CARTESIAN_POINT('Ctrl Pts',(0.900000001879218,-1.28788040990034,
0.605337476551906));
#12893=CARTESIAN_POINT('Ctrl Pts',(0.709864288600121,-1.28346276435313,
0.605340219076093));
#12894=CARTESIAN_POINT('Ctrl Pts',(0.519721397561595,-1.27909449722757,
0.60534313598158));
#12895=CARTESIAN_POINT('Ctrl Pts',(0.32957180616905,-1.2747428754212,0.605346305703265));
#12896=CARTESIAN_POINT('',(0.331856371369201,-1.17491202962433,0.7));
#12897=CARTESIAN_POINT('Origin',(0.331856371539144,-1.1749120296049,0.6));
#12898=CARTESIAN_POINT('Ctrl Pts',(0.900000000000328,-1.18799600975363,
0.7));
#12899=CARTESIAN_POINT('Ctrl Pts',(0.71062007065371,-1.18359647108512,0.7));
#12900=CARTESIAN_POINT('Ctrl Pts',(0.521238702715143,-1.17924592340069,
0.7));
#12901=CARTESIAN_POINT('Ctrl Pts',(0.331856371369203,-1.17491202960101,
0.7));
#12902=CARTESIAN_POINT('Origin',(6.87409734069396,-2.22251806091942E-16,
0.7));
#12903=CARTESIAN_POINT('',(0.331856371879032,1.17491202961268,0.7));
#12904=CARTESIAN_POINT('',(0.331856371369201,-0.75,0.7));
#12905=CARTESIAN_POINT('Ctrl Pts',(0.331856371879031,1.17491202961268,0.7));
#12906=CARTESIAN_POINT('Ctrl Pts',(0.521238703055026,1.1792459234085,0.7));
#12907=CARTESIAN_POINT('Ctrl Pts',(0.710620070823648,1.18359647108907,0.7));
#12908=CARTESIAN_POINT('Ctrl Pts',(0.900000000000325,1.18799600975363,0.7));
#12909=CARTESIAN_POINT('Ctrl Pts',(0.297857073289265,1.30643674434242,-1.84041299971672E-5));
#12910=CARTESIAN_POINT('Ctrl Pts',(0.30797052782623,1.29586163793935,0.201769818898405));
#12911=CARTESIAN_POINT('Ctrl Pts',(0.318084017341667,1.28528653282265,0.403558040242397));
#12912=CARTESIAN_POINT('Ctrl Pts',(0.328197542344371,1.27471142901691,0.605346259877786));
#12913=CARTESIAN_POINT('Ctrl Pts',(0.49855879921793,1.31100715551957,-1.17746012218085E-5));
#12914=CARTESIAN_POINT('Ctrl Pts',(0.50835067796626,1.30043204942878,0.201776459067662));
#12915=CARTESIAN_POINT('Ctrl Pts',(0.518142591787414,1.28985694462549,0.403564691103219));
#12916=CARTESIAN_POINT('Ctrl Pts',(0.527934541191015,1.27928184113928,0.60535292148228));
#12917=CARTESIAN_POINT('Ctrl Pts',(0.699273108318888,1.31559634352235,-5.70013621459206E-6));
#12918=CARTESIAN_POINT('Ctrl Pts',(0.708743431409089,1.3050212387088,0.201782543309265));
#12919=CARTESIAN_POINT('Ctrl Pts',(0.718213789762737,1.29444613519316,0.403570785168614));
#12920=CARTESIAN_POINT('Ctrl Pts',(0.727684183892215,1.28387103300524,0.605359025419352));
#12921=CARTESIAN_POINT('Ctrl Pts',(0.9,1.32024227787037,-6.93889390390723E-18));
#12922=CARTESIAN_POINT('Ctrl Pts',(0.909148787559144,1.30966717532775,0.201788252648578));
#12923=CARTESIAN_POINT('Ctrl Pts',(0.918297610668582,1.29909207410301,0.403576503755731));
#12924=CARTESIAN_POINT('Ctrl Pts',(0.927446469845411,1.28851697422136,0.605364753299355));
#12925=CARTESIAN_POINT('',(0.329571806169048,1.2747428754212,0.605346305703265));
#12926=CARTESIAN_POINT('Ctrl Pts',(0.900000001879216,1.28788040990034,0.605337476551906));
#12927=CARTESIAN_POINT('Ctrl Pts',(0.709864288600119,1.28346276435313,0.605340219076093));
#12928=CARTESIAN_POINT('Ctrl Pts',(0.519721397561593,1.27909449722757,0.60534313598158));
#12929=CARTESIAN_POINT('Ctrl Pts',(0.329571806169048,1.2747428754212,0.605346305703265));
#12930=CARTESIAN_POINT('Ctrl Pts',(0.329571806169048,1.2747428754212,0.605346305703265));
#12931=CARTESIAN_POINT('Ctrl Pts',(0.319000553694994,1.28530712634462,0.403564200350134));
#12932=CARTESIAN_POINT('Ctrl Pts',(0.308429283449307,1.29587142805659,0.201782098465301));
#12933=CARTESIAN_POINT('Ctrl Pts',(0.297857995688647,1.306435779838,6.03900610074426E-17));
#12934=CARTESIAN_POINT('Ctrl Pts',(0.331856371369201,1.17491202960101,0.7));
#12935=CARTESIAN_POINT('Ctrl Pts',(0.522011847238246,1.17926361631973,0.7));
#12936=CARTESIAN_POINT('Ctrl Pts',(0.712166351817729,1.18363199317816,0.7));
#12937=CARTESIAN_POINT('Ctrl Pts',(0.902319404079528,1.18804989493878,0.7));
#12938=CARTESIAN_POINT('Ctrl Pts',(0.331195161244124,1.20380556524924,0.7));
#12939=CARTESIAN_POINT('Ctrl Pts',(0.521348914609443,1.20815772874132,0.700000022626678));
#12940=CARTESIAN_POINT('Ctrl Pts',(0.711500071980329,1.21252656425213,0.69999998041973));
#12941=CARTESIAN_POINT('Ctrl Pts',(0.901648075315331,1.21694488185794,0.7));
#12942=CARTESIAN_POINT('Ctrl Pts',(0.330048718948197,1.25390275839508,0.676667306001616));
#12943=CARTESIAN_POINT('Ctrl Pts',(0.52019950796711,1.25825584722226,0.676666267597973));
#12944=CARTESIAN_POINT('Ctrl Pts',(0.710344780071469,1.26262550764723,0.676665329845182));
#12945=CARTESIAN_POINT('Ctrl Pts',(0.900484091294292,1.26704448261357,0.676664431332698));
#12946=CARTESIAN_POINT('Ctrl Pts',(0.329598318905018,1.27358432286302,0.626991130804315));
#12947=CARTESIAN_POINT('Ctrl Pts',(0.519747959090446,1.27793661492756,0.62698844527393));
#12948=CARTESIAN_POINT('Ctrl Pts',(0.709890987426057,1.28230548388611,0.626985988983916));
#12949=CARTESIAN_POINT('Ctrl Pts',(0.900026875890748,1.28672371253673,0.626983665342106));
#12950=CARTESIAN_POINT('Ctrl Pts',(0.329571806169048,1.2747428754212,0.605346305703265));
#12951=CARTESIAN_POINT('Ctrl Pts',(0.519721397561593,1.27909449722757,0.60534313598158));
#12952=CARTESIAN_POINT('Ctrl Pts',(0.709864288600119,1.28346276435313,0.605340219076093));
#12953=CARTESIAN_POINT('Ctrl Pts',(0.900000001879216,1.28788040990034,0.605337476551906));
#12954=CARTESIAN_POINT('Origin',(0.331856371369202,1.17491202960101,0.6));
#12955=CARTESIAN_POINT('Origin',(0.331856371369202,1.17491202960101,0.6));
#12956=CARTESIAN_POINT('Origin',(0.331856371369201,1.17491202960879,0.6));
#12957=CARTESIAN_POINT('Origin',(0.331856371369202,1.17491202960101,0.6));
#12958=CARTESIAN_POINT('Origin',(12.8681436286308,1.83274446434879,0.6));
#12959=CARTESIAN_POINT('Origin',(12.8681436286308,1.83274446434879,0.6));
#12960=CARTESIAN_POINT('',(12.9680065821063,1.83274446434879,0.605233595624294));
#12961=CARTESIAN_POINT('Origin',(12.8681436286308,1.83274446434879,0.6));
#12962=CARTESIAN_POINT('Origin',(12.8681436286308,1.83274446434879,0.6));
#12963=CARTESIAN_POINT('Origin',(0.331856371369201,-1.17491202960101,0.6));
#12964=CARTESIAN_POINT('Origin',(0.331856371369201,-1.17491202960101,0.6));
#12965=CARTESIAN_POINT('Origin',(0.331856371369201,-1.17491202960101,0.6));
#12966=CARTESIAN_POINT('Origin',(0.331856371369201,-0.75,0.6));
#12967=CARTESIAN_POINT('Ctrl Pts',(0.297750759617602,-1.30654294555098,
-0.00204689530870639));
#12968=CARTESIAN_POINT('Ctrl Pts',(0.308357792853923,-1.29594287152607,
0.200417501569666));
#12969=CARTESIAN_POINT('Ctrl Pts',(0.318964808457496,-1.28534284790734,
0.40288190189057));
#12970=CARTESIAN_POINT('Ctrl Pts',(0.329571806169048,-1.2747428754212,0.605346305703266));
#12971=CARTESIAN_POINT('Ctrl Pts',(0.268364475985512,-1.30579334864515,
-0.000546070465277405));
#12972=CARTESIAN_POINT('Ctrl Pts',(0.278972236061358,-1.29519218153762,
0.201918231169276));
#12973=CARTESIAN_POINT('Ctrl Pts',(0.289579970322816,-1.28459115545203,
0.404382541571378));
#12974=CARTESIAN_POINT('Ctrl Pts',(0.300187702091134,-1.27399007937578,
0.606846849214128));
#12975=CARTESIAN_POINT('Ctrl Pts',(0.217994620733579,-1.28028753054242,
0.000758348866131992));
#12976=CARTESIAN_POINT('Ctrl Pts',(0.228604439653725,-1.26968580576698,
0.203222517770204));
#12977=CARTESIAN_POINT('Ctrl Pts',(0.239214264875756,-1.259084092946,0.405686686833815));
#12978=CARTESIAN_POINT('Ctrl Pts',(0.24982407554016,-1.24848245399652,0.608150860486448));
#12979=CARTESIAN_POINT('Ctrl Pts',(0.200221638751335,-1.22875730734246,
-0.00100806500432267));
#12980=CARTESIAN_POINT('Ctrl Pts',(0.210832346469089,-1.21815680658782,
0.201456130081263));
#12981=CARTESIAN_POINT('Ctrl Pts',(0.221443027663539,-1.20755634130466,
0.403920328365886));
#12982=CARTESIAN_POINT('Ctrl Pts',(0.232053735729819,-1.1969559383274,0.606384528499152));
#12983=CARTESIAN_POINT('Ctrl Pts',(0.200161316008396,-1.20671181983024,
-0.00215909150772397));
#12984=CARTESIAN_POINT('Ctrl Pts',(0.21077201649647,-1.19611183845239,0.200305134857769));
#12985=CARTESIAN_POINT('Ctrl Pts',(0.221382717124246,-1.18551190812967,
0.402769363888924));
#12986=CARTESIAN_POINT('Ctrl Pts',(0.231993417893744,-1.17491202960101,
0.605233595624295));
#12987=CARTESIAN_POINT('Origin',(12.8681436286308,-1.83274446434879,0.6));
#12988=CARTESIAN_POINT('',(12.9680065821063,-1.83274446434879,0.605233595624295));
#12989=CARTESIAN_POINT('Origin',(12.8681436286308,-1.83274446434879,0.6));
#12990=CARTESIAN_POINT('Origin',(12.8681436286308,-1.83274446434879,0.6));
#12991=CARTESIAN_POINT('Origin',(12.8681436286308,1.1,0.6));
#12992=CARTESIAN_POINT('',(12.9680065821063,1.1,0.605233595624295));
#12993=CARTESIAN_POINT('Ctrl Pts',(12.9998428721614,-1.86475648739599,-0.00223900654757928));
#12994=CARTESIAN_POINT('Ctrl Pts',(12.9892307746816,-1.85408610159386,0.200251876006837));
#12995=CARTESIAN_POINT('Ctrl Pts',(12.9786186779927,-1.84341542867022,0.402742743472647));
#12996=CARTESIAN_POINT('Ctrl Pts',(12.9680065821063,-1.83274446434879,0.605233595624296));
#12997=CARTESIAN_POINT('Ctrl Pts',(12.9997989521977,-1.88070362541494,-0.00140096371806573));
#12998=CARTESIAN_POINT('Ctrl Pts',(12.9891868560404,-1.87003481788623,0.2010900171988));
#12999=CARTESIAN_POINT('Ctrl Pts',(12.9785747412344,-1.85936572080465,0.403580981971657));
#13000=CARTESIAN_POINT('Ctrl Pts',(12.967962646681,-1.84869634914788,0.606071933479074));
#13001=CARTESIAN_POINT('Ctrl Pts',(12.9919061104719,-1.91252097257855,-0.00013797468654593));
#13002=CARTESIAN_POINT('Ctrl Pts',(12.9812924311808,-1.9018552985481,0.202353118580234));
#13003=CARTESIAN_POINT('Ctrl Pts',(12.970678744243,-1.89118929884075,0.404844194499128));
#13004=CARTESIAN_POINT('Ctrl Pts',(12.9600650516023,-1.88052308923615,0.607335259545336));
#13005=CARTESIAN_POINT('Ctrl Pts',(12.9539932318948,-1.95585643963679,0.000158685530800887));
#13006=CARTESIAN_POINT('Ctrl Pts',(12.9433725220626,-1.94519261899951,0.202649549046396));
#13007=CARTESIAN_POINT('Ctrl Pts',(12.9327517623504,-1.93452853669393,0.40514039680648));
#13008=CARTESIAN_POINT('Ctrl Pts',(12.9221309734579,-1.92386419524738,0.607631230057729));
#13009=CARTESIAN_POINT('Ctrl Pts',(12.9129235702791,-1.96658826742031,-0.00142816374191492));
#13010=CARTESIAN_POINT('Ctrl Pts',(12.9022969271978,-1.95592037993921,0.201062184830579));
#13011=CARTESIAN_POINT('Ctrl Pts',(12.891670251582,-1.94525202616943,0.403552507423554));
#13012=CARTESIAN_POINT('Ctrl Pts',(12.8810434760214,-1.93458357684419,0.60604282089977));
#13013=CARTESIAN_POINT('Ctrl Pts',(12.8891437477602,-1.96405813112492,-0.00280773857265357));
#13014=CARTESIAN_POINT('Ctrl Pts',(12.8785151960038,-1.95338599020215,0.199682283294402));
#13015=CARTESIAN_POINT('Ctrl Pts',(12.8678865709412,-1.94271355010484,0.402172286243574));
#13016=CARTESIAN_POINT('Ctrl Pts',(12.8572578715866,-1.93204080633595,0.604662269998931));
#13017=CARTESIAN_POINT('Ctrl Pts',(12.9997255308004,-1.86463850151065,-4.9439619065339E-17));
#13018=CARTESIAN_POINT('Ctrl Pts',(12.9891525471135,-1.85400744222428,0.201744546927532));
#13019=CARTESIAN_POINT('Ctrl Pts',(12.9785795642115,-1.84337609791338,0.403489078876654));
#13020=CARTESIAN_POINT('Ctrl Pts',(12.9680065821063,-1.83274446434879,0.605233595624296));
#13021=CARTESIAN_POINT('Ctrl Pts',(12.8891409639924,1.96405533594058,-0.00275470357795049));
#13022=CARTESIAN_POINT('Ctrl Pts',(12.8785133401458,1.95338412669368,0.199717639954231));
#13023=CARTESIAN_POINT('Ctrl Pts',(12.8678856430057,1.9427126183241,0.402189964571813));
#13024=CARTESIAN_POINT('Ctrl Pts',(12.8572578715866,1.93204080633595,0.604662269998929));
#13025=CARTESIAN_POINT('Ctrl Pts',(12.9049941793403,1.96574209420267,-0.00183498696757459));
#13026=CARTESIAN_POINT('Ctrl Pts',(12.8943678341644,1.95507368670196,0.20063757283533));
#13027=CARTESIAN_POINT('Ctrl Pts',(12.8837414238008,1.94440496992476,0.403110113573296));
#13028=CARTESIAN_POINT('Ctrl Pts',(12.8731149412098,1.93373598667478,0.605582637266155));
#13029=CARTESIAN_POINT('Ctrl Pts',(12.9374710816243,1.9613461313261,-0.000364592700753267));
#13030=CARTESIAN_POINT('Ctrl Pts',(12.9268487371951,1.95068187676899,0.202108391447626));
#13031=CARTESIAN_POINT('Ctrl Pts',(12.9162262930262,1.94001732715406,0.404581355450702));
#13032=CARTESIAN_POINT('Ctrl Pts',(12.9056038462248,1.92935253789361,0.607054307450502));
#13033=CARTESIAN_POINT('Ctrl Pts',(12.9846523118271,1.92834870343354,0.000369250346899581));
#13034=CARTESIAN_POINT('Ctrl Pts',(12.974038022963,1.91768545846127,0.202842678583437));
#13035=CARTESIAN_POINT('Ctrl Pts',(12.9634237233674,1.90702194269714,0.405316092420461));
#13036=CARTESIAN_POINT('Ctrl Pts',(12.9528094065597,1.89635817580376,0.607789492622546));
#13037=CARTESIAN_POINT('Ctrl Pts',(12.9997742127558,1.88867440031858,-0.000928907044737527));
#13038=CARTESIAN_POINT('Ctrl Pts',(12.9891630904765,1.8780073281596,0.201544447891303));
#13039=CARTESIAN_POINT('Ctrl Pts',(12.9785517991681,1.86733992038445,0.404017776344753));
#13040=CARTESIAN_POINT('Ctrl Pts',(12.9679406789684,1.85667229154743,0.606491102406462));
#13041=CARTESIAN_POINT('Ctrl Pts',(12.9998400927033,1.86475369267134,-0.00218597132744988));
#13042=CARTESIAN_POINT('Ctrl Pts',(12.9892289217097,1.85408423839396,0.200287232817622));
#13043=CARTESIAN_POINT('Ctrl Pts',(12.9786177515068,1.84341449704483,0.402760421876702));
#13044=CARTESIAN_POINT('Ctrl Pts',(12.9680065821063,1.83274446434879,0.605233595624294));
#13045=CARTESIAN_POINT('Ctrl Pts',(12.9680065821063,1.83274446434879,0.605233595624294));
#13046=CARTESIAN_POINT('Ctrl Pts',(12.9785795642115,1.84337609791338,0.403489078876654));
#13047=CARTESIAN_POINT('Ctrl Pts',(12.9891525471135,1.85400744222428,0.201744546927532));
#13048=CARTESIAN_POINT('Ctrl Pts',(12.9997255308004,1.86463850151065,1.86916454536501E-16));
#13049=CARTESIAN_POINT('Ctrl Pts',(12.6,1.80383022254432,0.7));
#13050=CARTESIAN_POINT('Ctrl Pts',(12.6893984576578,1.8133105623702,0.7));
#13051=CARTESIAN_POINT('Ctrl Pts',(12.7787800350189,1.82294762441299,0.7));
#13052=CARTESIAN_POINT('Ctrl Pts',(12.8681436286308,1.83274446434879,0.7));
#13053=CARTESIAN_POINT('Ctrl Pts',(12.5969393303222,1.83269196733649,0.7));
#13054=CARTESIAN_POINT('Ctrl Pts',(12.686303642571,1.84217134991284,0.700000098415946));
#13055=CARTESIAN_POINT('Ctrl Pts',(12.7756511334299,1.85180730951691,0.699999896874207));
#13056=CARTESIAN_POINT('Ctrl Pts',(12.8649798835675,1.86160311979107,0.7));
#13057=CARTESIAN_POINT('Ctrl Pts',(12.5916356538948,1.88270499442536,0.67643906321291));
#13058=CARTESIAN_POINT('Ctrl Pts',(12.6809412203008,1.89218243450198,0.676434576658958));
#13059=CARTESIAN_POINT('Ctrl Pts',(12.7702288461642,1.90181652272411,0.676430055978541));
#13060=CARTESIAN_POINT('Ctrl Pts',(12.8594976525144,1.91161025179704,0.676425356750174));
#13061=CARTESIAN_POINT('Ctrl Pts',(12.58957419749,1.90214427893475,0.626447702441804));
#13062=CARTESIAN_POINT('Ctrl Pts',(12.6788572782758,1.91161594713488,0.626436135819418));
#13063=CARTESIAN_POINT('Ctrl Pts',(12.7681225846323,1.92124403769089,0.626424372515079));
#13064=CARTESIAN_POINT('Ctrl Pts',(12.8573684983393,1.93103170500986,0.626412260100396));
#13065=CARTESIAN_POINT('Ctrl Pts',(12.5894662143615,1.90316254677271,0.604704117718382));
#13066=CARTESIAN_POINT('Ctrl Pts',(12.6787484942245,1.91263121188366,0.60469048808123));
#13067=CARTESIAN_POINT('Ctrl Pts',(12.7680127446979,1.92225628370762,0.604676541242762));
#13068=CARTESIAN_POINT('Ctrl Pts',(12.8572578715866,1.93204080633595,0.60466226999893));
#13069=CARTESIAN_POINT('Ctrl Pts',(0.200160815981423,1.20671231935208,-0.00216863259073552));
#13070=CARTESIAN_POINT('Ctrl Pts',(0.21077168314515,1.19611217146534,0.200298774135678));
#13071=CARTESIAN_POINT('Ctrl Pts',(0.221382550448584,1.18551207463533,0.402766183527835));
#13072=CARTESIAN_POINT('Ctrl Pts',(0.231993417893744,1.17491202960101,0.605233595624295));
#13073=CARTESIAN_POINT('Ctrl Pts',(0.200241246305444,1.23610630273461,-0.000633930584249493));
#13074=CARTESIAN_POINT('Ctrl Pts',(0.210852138766318,1.22550544237485,0.201833432539687));
#13075=CARTESIAN_POINT('Ctrl Pts',(0.221462948692539,1.21490467236247,0.404300804744641));
#13076=CARTESIAN_POINT('Ctrl Pts',(0.232073841675177,1.20430390790287,0.60676817279077));
#13077=CARTESIAN_POINT('Ctrl Pts',(0.224595236946023,1.28704077752974,0.000756396927320467));
#13078=CARTESIAN_POINT('Ctrl Pts',(0.235204871724134,1.27643877611169,0.203223757667495));
#13079=CARTESIAN_POINT('Ctrl Pts',(0.245814524913363,1.26583679641595,0.405691118453359));
#13080=CARTESIAN_POINT('Ctrl Pts',(0.256424148042823,1.25523487973404,0.608158484046399));
#13081=CARTESIAN_POINT('Ctrl Pts',(0.275710547013829,1.30598124743532,-0.000930817763883136));
#13082=CARTESIAN_POINT('Ctrl Pts',(0.286318282165364,1.29538020346814,0.201536689442792));
#13083=CARTESIAN_POINT('Ctrl Pts',(0.296926023167072,1.2847792285374,0.404004199876323));
#13084=CARTESIAN_POINT('Ctrl Pts',(0.307533728110612,1.27417827838713,0.606471713336412));
#13085=CARTESIAN_POINT('Ctrl Pts',(0.297750259763447,1.30654344507719,-0.0020564363997533));
#13086=CARTESIAN_POINT('Ctrl Pts',(0.308357459618374,1.29594320454196,0.200411140842193));
#13087=CARTESIAN_POINT('Ctrl Pts',(0.318964641840002,1.28534301441448,0.402878721526778));
#13088=CARTESIAN_POINT('Ctrl Pts',(0.329571806169048,1.2747428754212,0.605346305703265));
#13089=CARTESIAN_POINT('Origin',(13.0002740930491,2.2,-0.0104671912485888));
#13090=CARTESIAN_POINT('Origin',(0.331856371369202,1.17491202960101,0.6));
#13091=CARTESIAN_POINT('',(0.331856371879032,1.17491202961268,0.9));
#13092=CARTESIAN_POINT('',(0.0322675109428289,1.17491202960101,0.615700786872883));
#13093=CARTESIAN_POINT('Origin',(0.331856371369201,1.17491202962433,0.6));
#13094=CARTESIAN_POINT('',(0.325002675768741,1.47440456706157,0.616038917109795));
#13095=CARTESIAN_POINT('Origin',(0.331856371369202,1.17491202960101,0.6));
#13096=CARTESIAN_POINT('Origin',(0.331856371369201,1.17491202960101,0.6));
#13097=CARTESIAN_POINT('Origin',(12.8681436286308,1.83274446434879,0.6));
#13098=CARTESIAN_POINT('',(12.8681436286308,1.83274446434879,0.9));
#13099=CARTESIAN_POINT('',(12.8354863574981,2.13063349031027,0.613986809996789));
#13100=CARTESIAN_POINT('Origin',(12.8681436286308,1.83274446434879,0.6));
#13101=CARTESIAN_POINT('',(13.1677324890572,1.83274446434879,0.615700786872883));
#13102=CARTESIAN_POINT('Origin',(12.8681436286308,1.83274446434879,0.6));
#13103=CARTESIAN_POINT('Origin',(12.8681436286308,1.83274446434879,0.6));
#13104=CARTESIAN_POINT('Origin',(0.331856371369201,-1.17491202960101,0.6));
#13105=CARTESIAN_POINT('',(0.331856371369201,-1.17491202962433,0.9));
#13106=CARTESIAN_POINT('',(0.325002675768743,-1.47440456706157,0.616038917109795));
#13107=CARTESIAN_POINT('Origin',(0.331856371879032,-1.17491202961268,0.6));
#13108=CARTESIAN_POINT('',(0.0322675109428289,-1.17491202960101,0.615700786872884));
#13109=CARTESIAN_POINT('Origin',(0.331856371369201,-1.17491202960101,0.6));
#13110=CARTESIAN_POINT('Origin',(0.331856371369201,-1.17491202960101,0.6));
#13111=CARTESIAN_POINT('Origin',(0.331856371369201,-0.75,0.6));
#13112=CARTESIAN_POINT('',(0.0322675109428289,-0.75,0.615700786872883));
#13113=CARTESIAN_POINT('',(0.331856371369201,-0.75,0.9));
#13114=CARTESIAN_POINT('Ctrl Pts',(0.292429673212981,-1.5069793045954,-0.00614074949474724));
#13115=CARTESIAN_POINT('Ctrl Pts',(0.303287396789886,-1.49612100698918,
0.201252467440773));
#13116=CARTESIAN_POINT('Ctrl Pts',(0.314145064588525,-1.48526276089333,
0.408645689616972));
#13117=CARTESIAN_POINT('Ctrl Pts',(0.325002675768741,-1.47440456706157,
0.616038917109795));
#13118=CARTESIAN_POINT('Ctrl Pts',(0.204270663953122,-1.50473074636003,
-0.00163825452108868));
#13119=CARTESIAN_POINT('Ctrl Pts',(0.215130619942527,-1.49386909866124,
0.205754670272474));
#13120=CARTESIAN_POINT('Ctrl Pts',(0.225990497234893,-1.48300775583971,
0.413147615201549));
#13121=CARTESIAN_POINT('Ctrl Pts',(0.236850363534999,-1.47214617892531,
0.620540547642382));
#13122=CARTESIAN_POINT('Ctrl Pts',(0.0531014592841718,-1.42831231122466,
0.00228331220810075));
#13123=CARTESIAN_POINT('Ctrl Pts',(0.0639677431943945,-1.41744892560022,
0.209675827753147));
#13124=CARTESIAN_POINT('Ctrl Pts',(0.0748340498672138,-1.40658548887187,
0.417068339030394));
#13125=CARTESIAN_POINT('Ctrl Pts',(0.0857003072238147,-1.3957221574093,
0.624460858243749));
#13126=CARTESIAN_POINT('Ctrl Pts',(-0.000158492362241063,-1.27362248439808,
-0.0030242144278773));
#13127=CARTESIAN_POINT('Ctrl Pts',(0.0107105192099893,-1.2627628846508,
0.204368383073371));
#13128=CARTESIAN_POINT('Ctrl Pts',(0.0215794523842628,-1.25190326350425,
0.411760983371354));
#13129=CARTESIAN_POINT('Ctrl Pts',(0.0324484644510542,-1.24104375578019,
0.619153585497454));
#13130=CARTESIAN_POINT('Ctrl Pts',(-0.000339460947516079,-1.20748590713937,
-0.00647730073969574));
#13131=CARTESIAN_POINT('Ctrl Pts',(0.0105295295353408,-1.19662789414299,
0.200915392321314));
#13132=CARTESIAN_POINT('Ctrl Pts',(0.0213985201647323,-1.18576993469886,
0.408308088178364));
#13133=CARTESIAN_POINT('Ctrl Pts',(0.032267510942829,-1.17491202960101,
0.615700786872884));
#13134=CARTESIAN_POINT('Ctrl Pts',(0.292751161823634,-1.50665779898694,
4.33680868994202E-17));
#13135=CARTESIAN_POINT('Ctrl Pts',(0.30350172143464,-1.49590667092872,0.205346300540216));
#13136=CARTESIAN_POINT('Ctrl Pts',(0.314252226354851,-1.48515559337638,
0.410692606218909));
#13137=CARTESIAN_POINT('Ctrl Pts',(0.325002675768741,-1.47440456706157,
0.616038917109795));
#13138=CARTESIAN_POINT('Ctrl Pts',(0.032267510942829,-1.17491202960101,
0.615700786872884));
#13139=CARTESIAN_POINT('Ctrl Pts',(0.021511673816962,-1.18565689645617,
0.410467188483275));
#13140=CARTESIAN_POINT('Ctrl Pts',(0.0107558368367201,-1.19640181653194,
0.205233592872363));
#13141=CARTESIAN_POINT('Ctrl Pts',(-2.19605150036939E-16,-1.20714678905882,
1.11889664200504E-16));
#13142=CARTESIAN_POINT('Origin',(12.8681436286308,-1.83274446434879,0.6));
#13143=CARTESIAN_POINT('',(13.1677324890572,-1.83274446434879,0.615700786872883));
#13144=CARTESIAN_POINT('',(12.8354863574981,-2.13063349031027,0.613986809996789));
#13145=CARTESIAN_POINT('Origin',(12.8681436286308,-1.83274446434879,0.6));
#13146=CARTESIAN_POINT('',(12.8681436286308,-1.83274446434879,0.9));
#13147=CARTESIAN_POINT('Origin',(12.8681436286308,-1.83274446434879,0.6));
#13148=CARTESIAN_POINT('Origin',(12.8681436286308,-1.83274446434879,0.6));
#13149=CARTESIAN_POINT('Origin',(12.8681436286308,1.1,0.6));
#13150=CARTESIAN_POINT('',(13.1677324890572,1.1,0.615700786872883));
#13151=CARTESIAN_POINT('',(12.8681436286308,1.1,0.9));
#13152=CARTESIAN_POINT('Ctrl Pts',(12.8681436286308,-1.83274446434879,0.9));
#13153=CARTESIAN_POINT('Ctrl Pts',(11.0848390724976,-1.63724259846481,0.9));
#13154=CARTESIAN_POINT('Ctrl Pts',(6.90843812479705,-1.33014681916253,0.9));
#13155=CARTESIAN_POINT('Ctrl Pts',(2.72316671642812,-1.22963564084767,0.9));
#13156=CARTESIAN_POINT('Ctrl Pts',(0.331856371369203,-1.17491202960101,
0.9));
#13157=CARTESIAN_POINT('Ctrl Pts',(12.8586523934408,-1.91932043067563,0.9));
#13158=CARTESIAN_POINT('Ctrl Pts',(11.0774332085042,-1.7238803779394,0.89999435405169));
#13159=CARTESIAN_POINT('Ctrl Pts',(6.90489492800773,-1.41683381760594,0.900002805573959));
#13160=CARTESIAN_POINT('Ctrl Pts',(2.72111811994416,-1.31633797570969,0.90000078069347));
#13161=CARTESIAN_POINT('Ctrl Pts',(0.329872740993971,-1.26159263654569,
0.9));
#13162=CARTESIAN_POINT('Ctrl Pts',(12.8422006781022,-2.06938763738452,0.829321796184829));
#13163=CARTESIAN_POINT('Ctrl Pts',(11.0645720435655,-1.87407163985848,0.829602081442736));
#13164=CARTESIAN_POINT('Ctrl Pts',(6.89876476423634,-1.56711486110062,0.829953500700133));
#13165=CARTESIAN_POINT('Ctrl Pts',(2.71756729604702,-1.46664725828863,0.829952661937692));
#13166=CARTESIAN_POINT('Ctrl Pts',(0.326433810179884,-1.41186690836963,
0.829991693349937));
#13167=CARTESIAN_POINT('Ctrl Pts',(12.8358182377562,-2.12760618633201,0.679236780301187));
#13168=CARTESIAN_POINT('Ctrl Pts',(11.0595580661442,-1.93265366192027,0.679962478070753));
#13169=CARTESIAN_POINT('Ctrl Pts',(6.89634818471837,-1.62613750062048,0.680874066334139));
#13170=CARTESIAN_POINT('Ctrl Pts',(2.71617242066404,-1.52567909229178,0.680871998075852));
#13171=CARTESIAN_POINT('Ctrl Pts',(0.325082213976654,-1.47092890938704,
0.680973392412944));
#13172=CARTESIAN_POINT('Ctrl Pts',(12.8354863574981,-2.13063349031027,0.613986809996789));
#13173=CARTESIAN_POINT('Ctrl Pts',(11.0592740266891,-1.93586902238569,0.614841183901826));
#13174=CARTESIAN_POINT('Ctrl Pts',(6.89620783868867,-1.62958780289117,0.615922665333222));
#13175=CARTESIAN_POINT('Ctrl Pts',(2.71609101918193,-1.52912950204849,0.615919334096661));
#13176=CARTESIAN_POINT('Ctrl Pts',(0.325002675768742,-1.47440456706157,
0.616038917109795));
#13177=CARTESIAN_POINT('Ctrl Pts',(0.325002675768742,-1.47440456706157,
0.616038917109795));
#13178=CARTESIAN_POINT('Ctrl Pts',(2.71609101918193,-1.52912950204849,0.615919334096661));
#13179=CARTESIAN_POINT('Ctrl Pts',(6.89620783868867,-1.62958780289117,0.615922665333222));
#13180=CARTESIAN_POINT('Ctrl Pts',(11.0592740266891,-1.93586902238569,0.614841183901826));
#13181=CARTESIAN_POINT('Ctrl Pts',(12.8354863574981,-2.13063349031027,0.613986809996789));
#13182=CARTESIAN_POINT('Ctrl Pts',(12.8681436286308,-1.83274446434879,0.9));
#13183=CARTESIAN_POINT('Ctrl Pts',(11.0848390724976,-1.63724259846481,0.9));
#13184=CARTESIAN_POINT('Ctrl Pts',(6.90843812479705,-1.33014681916253,0.9));
#13185=CARTESIAN_POINT('Ctrl Pts',(2.72316671642812,-1.22963564084767,0.9));
#13186=CARTESIAN_POINT('Ctrl Pts',(0.331856371369203,-1.17491202960101,
0.9));
#13187=CARTESIAN_POINT('Ctrl Pts',(13.2003520234216,-1.86554403325358,-0.00671700702553119));
#13188=CARTESIAN_POINT('Ctrl Pts',(13.1894788444661,-1.85461114646479,0.200755606855839));
#13189=CARTESIAN_POINT('Ctrl Pts',(13.1786056663403,-1.84367795836273,0.40822820490283));
#13190=CARTESIAN_POINT('Ctrl Pts',(13.1677324890572,-1.83274446434879,0.615700786872884));
#13191=CARTESIAN_POINT('Ctrl Pts',(13.200220264666,-1.91338509859121,-0.00420290020003313));
#13192=CARTESIAN_POINT('Ctrl Pts',(13.1893470894366,-1.90245705934317,0.203270015787334));
#13193=CARTESIAN_POINT('Ctrl Pts',(13.1784738563058,-1.89152871992859,0.410742913234898));
#13194=CARTESIAN_POINT('Ctrl Pts',(13.1676006827814,-1.88060011874606,0.61821580043722));
#13195=CARTESIAN_POINT('Ctrl Pts',(13.1765676699515,-2.00888806967359,-0.000409897060868941));
#13196=CARTESIAN_POINT('Ctrl Pts',(13.1656896254949,-1.99796966505382,0.207063364242462));
#13197=CARTESIAN_POINT('Ctrl Pts',(13.1548115799789,-1.98705090404177,0.414536607525659));
#13198=CARTESIAN_POINT('Ctrl Pts',(13.1439334900924,-1.97613202744891,0.622009843787749));
#13199=CARTESIAN_POINT('Ctrl Pts',(13.0627995670833,-2.13884429305335,0.000475886042502645));
#13200=CARTESIAN_POINT('Ctrl Pts',(13.0518999280859,-2.12793157960824,0.207948441605934));
#13201=CARTESIAN_POINT('Ctrl Pts',(13.041000104914,-2.11701865581933,0.415420978499924));
#13202=CARTESIAN_POINT('Ctrl Pts',(13.0301002136907,-2.10610551685206,0.62289350259018));
#13203=CARTESIAN_POINT('Ctrl Pts',(12.9395973356642,-2.17103883395928,-0.00428435975826336));
#13204=CARTESIAN_POINT('Ctrl Pts',(12.9286794517625,-2.16011362679945,0.203186612960554));
#13205=CARTESIAN_POINT('Ctrl Pts',(12.9177614752639,-2.14918756369419,0.410657536673191));
#13206=CARTESIAN_POINT('Ctrl Pts',(12.9068431708026,-2.13826180183499,0.618128462699307));
#13207=CARTESIAN_POINT('Ctrl Pts',(12.8682582931239,-2.16344935299393,-0.00842301254802964));
#13208=CARTESIAN_POINT('Ctrl Pts',(12.857334548107,-2.15251107312608,0.1990469563258));
#13209=CARTESIAN_POINT('Ctrl Pts',(12.8464105706338,-2.1415724540018,0.406516897309109));
#13210=CARTESIAN_POINT('Ctrl Pts',(12.8354863574981,-2.13063349031027,0.61398680999679));
#13211=CARTESIAN_POINT('Ctrl Pts',(13.2,-1.86519007666192,-2.60208521396521E-17));
#13212=CARTESIAN_POINT('Ctrl Pts',(13.1892441622028,-1.85437516893481,0.20523361119958));
#13213=CARTESIAN_POINT('Ctrl Pts',(13.1784883252177,-1.84355996631422,0.410467206902138));
#13214=CARTESIAN_POINT('Ctrl Pts',(13.1677324890572,-1.83274446434879,0.615700786872884));
#13215=CARTESIAN_POINT('Ctrl Pts',(12.8354863574981,-2.13063349031027,0.61398680999679));
#13216=CARTESIAN_POINT('Ctrl Pts',(12.8462627343229,-2.14142441807303,0.409324567403199));
#13217=CARTESIAN_POINT('Ctrl Pts',(12.8570388818204,-2.15221501053143,0.204662297274642));
#13218=CARTESIAN_POINT('Ctrl Pts',(12.8678148030684,-2.16300527278357,2.15973072759112E-16));
#13219=CARTESIAN_POINT('Ctrl Pts',(12.868249917342,2.16344096606744,-0.0082639349430893));
#13220=CARTESIAN_POINT('Ctrl Pts',(12.8573289641336,2.15250548166836,0.19915300804817));
#13221=CARTESIAN_POINT('Ctrl Pts',(12.8464077785869,2.14156965818488,0.406569923163064));
#13222=CARTESIAN_POINT('Ctrl Pts',(12.8354863574981,2.13063349031027,0.613986809996789));
#13223=CARTESIAN_POINT('Ctrl Pts',(12.9158092820513,2.16850062662823,-0.00550483257449158));
#13224=CARTESIAN_POINT('Ctrl Pts',(12.9048922561706,2.15757374897544,0.201912774743134));
#13225=CARTESIAN_POINT('Ctrl Pts',(12.8939750281693,2.14664650750606,0.409330354360154));
#13226=CARTESIAN_POINT('Ctrl Pts',(12.8830575663678,2.13571903132675,0.616747911798467));
#13227=CARTESIAN_POINT('Ctrl Pts',(13.0132876381743,2.15534286385676,-0.00108956416640176));
#13228=CARTESIAN_POINT('Ctrl Pts',(13.002382910411,2.14442874534411,0.206329347217122));
#13229=CARTESIAN_POINT('Ctrl Pts',(12.9914779109393,2.13351435475356,0.413748232116966));
#13230=CARTESIAN_POINT('Ctrl Pts',(12.9805728576194,2.12259976690609,0.621167106093357));
#13231=CARTESIAN_POINT('Ctrl Pts',(13.1547834649542,2.05631410774027,0.001107541479323));
#13232=CARTESIAN_POINT('Ctrl Pts',(13.1439034803964,2.04540309863889,0.208527817346591));
#13233=CARTESIAN_POINT('Ctrl Pts',(13.1330234810862,2.03449182132921,0.415948079627069));
#13234=CARTESIAN_POINT('Ctrl Pts',(13.1221434051731,2.0235803832085,0.623368331037722));
#13235=CARTESIAN_POINT('Ctrl Pts',(13.2001460482598,1.93729725403583,-0.00278676680844524));
#13236=CARTESIAN_POINT('Ctrl Pts',(13.1892758011844,1.92637447722781,0.204633283810596));
#13237=CARTESIAN_POINT('Ctrl Pts',(13.1784050234814,1.91545126126866,0.412053283701094));
#13238=CARTESIAN_POINT('Ctrl Pts',(13.1675347796435,1.9045279459447,0.619473307219386));
#13239=CARTESIAN_POINT('Ctrl Pts',(13.2003436864113,1.86553565046225,-0.00655792739252892));
#13240=CARTESIAN_POINT('Ctrl Pts',(13.1894732864596,1.85460555778322,0.200861659936414));
#13241=CARTESIAN_POINT('Ctrl Pts',(13.1786028873373,1.84367516394377,0.408281231439009));
#13242=CARTESIAN_POINT('Ctrl Pts',(13.1677324890572,1.83274446434879,0.615700786872883));
#13243=CARTESIAN_POINT('Ctrl Pts',(12.8678148030684,2.16300527278357,-3.77302356024956E-17));
#13244=CARTESIAN_POINT('Ctrl Pts',(12.8570388818204,2.15221501053142,0.204662297274639));
#13245=CARTESIAN_POINT('Ctrl Pts',(12.8462627343229,2.14142441807303,0.409324567403198));
#13246=CARTESIAN_POINT('Ctrl Pts',(12.8354863574981,2.13063349031027,0.613986809996789));
#13247=CARTESIAN_POINT('Ctrl Pts',(13.1677324890572,1.83274446434879,0.615700786872883));
#13248=CARTESIAN_POINT('Ctrl Pts',(13.1784883252177,1.84355996631422,0.410467206902138));
#13249=CARTESIAN_POINT('Ctrl Pts',(13.1892441622028,1.85437516893481,0.20523361119958));
#13250=CARTESIAN_POINT('Ctrl Pts',(13.2,1.86519007666192,9.4542429440736E-17));
#13251=CARTESIAN_POINT('Ctrl Pts',(0.3318563713692,1.17491202960101,0.9));
#13252=CARTESIAN_POINT('Ctrl Pts',(2.72316671642811,1.22963564084767,0.9));
#13253=CARTESIAN_POINT('Ctrl Pts',(6.90843812479704,1.33014681916253,0.9));
#13254=CARTESIAN_POINT('Ctrl Pts',(11.0848390724976,1.63724259846481,0.9));
#13255=CARTESIAN_POINT('Ctrl Pts',(12.8681436286308,1.83274446434879,0.9));
#13256=CARTESIAN_POINT('Ctrl Pts',(0.329872740993969,1.26159263654569,0.9));
#13257=CARTESIAN_POINT('Ctrl Pts',(2.72111811994415,1.31633797570969,0.90000078069347));
#13258=CARTESIAN_POINT('Ctrl Pts',(6.90489492800774,1.41683381760594,0.90000280557396));
#13259=CARTESIAN_POINT('Ctrl Pts',(11.0774332085042,1.7238803779394,0.89999435405169));
#13260=CARTESIAN_POINT('Ctrl Pts',(12.8586523934408,1.91932043067563,0.9));
#13261=CARTESIAN_POINT('Ctrl Pts',(0.326433810179882,1.41186690836963,0.829991693349937));
#13262=CARTESIAN_POINT('Ctrl Pts',(2.71756729604703,1.46664725828863,0.829952661937692));
#13263=CARTESIAN_POINT('Ctrl Pts',(6.89876476423633,1.56711486110062,0.829953500700133));
#13264=CARTESIAN_POINT('Ctrl Pts',(11.0645720435655,1.87407163985848,0.829602081442736));
#13265=CARTESIAN_POINT('Ctrl Pts',(12.8422006781022,2.06938763738452,0.829321796184828));
#13266=CARTESIAN_POINT('Ctrl Pts',(0.325082213976652,1.47092890938703,0.680973392412944));
#13267=CARTESIAN_POINT('Ctrl Pts',(2.71617242066403,1.52567909229178,0.680871998075852));
#13268=CARTESIAN_POINT('Ctrl Pts',(6.89634818471838,1.62613750062048,0.680874066334139));
#13269=CARTESIAN_POINT('Ctrl Pts',(11.0595580661442,1.93265366192027,0.679962478070753));
#13270=CARTESIAN_POINT('Ctrl Pts',(12.8358182377562,2.12760618633201,0.679236780301187));
#13271=CARTESIAN_POINT('Ctrl Pts',(0.32500267576874,1.47440456706157,0.616038917109795));
#13272=CARTESIAN_POINT('Ctrl Pts',(2.71609101918192,1.52912950204849,0.615919334096661));
#13273=CARTESIAN_POINT('Ctrl Pts',(6.89620783868868,1.62958780289117,0.615922665333222));
#13274=CARTESIAN_POINT('Ctrl Pts',(11.0592740266891,1.93586902238569,0.614841183901826));
#13275=CARTESIAN_POINT('Ctrl Pts',(12.8354863574981,2.13063349031027,0.613986809996789));
#13276=CARTESIAN_POINT('Ctrl Pts',(12.8354863574981,2.13063349031027,0.613986809996789));
#13277=CARTESIAN_POINT('Ctrl Pts',(11.0592740266891,1.93586902238569,0.614841183901826));
#13278=CARTESIAN_POINT('Ctrl Pts',(6.89620783868868,1.62958780289117,0.615922665333222));
#13279=CARTESIAN_POINT('Ctrl Pts',(2.71609101918192,1.52912950204849,0.615919334096661));
#13280=CARTESIAN_POINT('Ctrl Pts',(0.32500267576874,1.47440456706157,0.616038917109795));
#13281=CARTESIAN_POINT('Ctrl Pts',(0.331856371879031,1.17491202961268,0.900000000000001));
#13282=CARTESIAN_POINT('Ctrl Pts',(2.72316671676804,1.22963564085583,0.9));
#13283=CARTESIAN_POINT('Ctrl Pts',(6.90843812496665,1.330146819175,0.9));
#13284=CARTESIAN_POINT('Ctrl Pts',(11.0848390724976,1.63724259846481,0.9));
#13285=CARTESIAN_POINT('Ctrl Pts',(12.8681436286308,1.83274446434879,0.9));
#13286=CARTESIAN_POINT('Ctrl Pts',(-0.00034095850043725,1.20748740317979,
-0.0065058757516861));
#13287=CARTESIAN_POINT('Ctrl Pts',(0.0105285311667133,1.19662889149835,
0.200896342313063));
#13288=CARTESIAN_POINT('Ctrl Pts',(0.0213980209804115,1.18577043337405,
0.408298563174108));
#13289=CARTESIAN_POINT('Ctrl Pts',(0.0322675109428289,1.17491202960101,
0.615700786872884));
#13290=CARTESIAN_POINT('Ctrl Pts',(-9.96670524854573E-5,1.295669506487,
-0.00190176065173685));
#13291=CARTESIAN_POINT('Ctrl Pts',(0.0107698931059531,1.28480880908357,
0.205500324005663));
#13292=CARTESIAN_POINT('Ctrl Pts',(0.0216392211477595,1.27394827585187,
0.412902429485043));
#13293=CARTESIAN_POINT('Ctrl Pts',(0.0325087822871292,1.26308766450658,
0.62030451837231));
#13294=CARTESIAN_POINT('Ctrl Pts',(0.0728623575603101,1.44853010213391,
0.00227745497540766));
#13295=CARTESIAN_POINT('Ctrl Pts',(0.0837280751164453,1.43766588856392,
0.209679530627308));
#13296=CARTESIAN_POINT('Ctrl Pts',(0.0945938325013454,1.42680163888532,
0.41708160190494));
#13297=CARTESIAN_POINT('Ctrl Pts',(0.105459512942901,1.41593747613444,0.624483681552028));
#13298=CARTESIAN_POINT('Ctrl Pts',(0.226308920038025,1.50529438233544,-0.00279245331904538));
#13299=CARTESIAN_POINT('Ctrl Pts',(0.237168779176494,1.4944331215396,0.204610074087555));
#13300=CARTESIAN_POINT('Ctrl Pts',(0.248028678199983,1.48357195724705,0.412012604182119));
#13301=CARTESIAN_POINT('Ctrl Pts',(0.258888441593434,1.47271077595937,0.619415140009235));
#13302=CARTESIAN_POINT('Ctrl Pts',(0.292428177212438,1.50698080067503,-0.00616932457891824));
#13303=CARTESIAN_POINT('Ctrl Pts',(0.303286399461314,1.49612200437087,0.201233417384176));
#13304=CARTESIAN_POINT('Ctrl Pts',(0.314144565926839,1.48526325958177,0.408636164588429));
#13305=CARTESIAN_POINT('Ctrl Pts',(0.325002675768741,1.47440456706157,0.616038917109795));
#13306=CARTESIAN_POINT('Ctrl Pts',(1.62630325872826E-19,1.20714678905882,
-9.93129189996722E-17));
#13307=CARTESIAN_POINT('Ctrl Pts',(0.0107558368367203,1.19640181653194,
0.205233592872363));
#13308=CARTESIAN_POINT('Ctrl Pts',(0.0215116738169619,1.18565689645617,
0.410467188483274));
#13309=CARTESIAN_POINT('Ctrl Pts',(0.0322675109428289,1.17491202960101,
0.615700786872884));
#13310=CARTESIAN_POINT('Ctrl Pts',(0.325002675768741,1.47440456706157,0.616038917109795));
#13311=CARTESIAN_POINT('Ctrl Pts',(0.314252226354851,1.48515559337638,0.410692606218907));
#13312=CARTESIAN_POINT('Ctrl Pts',(0.30350172143464,1.49590667092872,0.205346300540215));
#13313=CARTESIAN_POINT('Ctrl Pts',(0.292751161823635,1.50665779898694,-1.27502175484295E-16));
#13314=CARTESIAN_POINT('Ctrl Pts',(12.8678148030684,-2.16300527278356,0.));
#13315=CARTESIAN_POINT('Ctrl Pts',(12.8575947095063,-2.15224352891768,0.205346305703265));
#13316=CARTESIAN_POINT('Ctrl Pts',(12.8473746159443,-2.14148178505179,0.41069261140653));
#13317=CARTESIAN_POINT('Ctrl Pts',(12.8371545223823,-2.13072004118591,0.616038917109795));
#13318=CARTESIAN_POINT('Ctrl Pts',(8.67612692265345,-1.70561506876628,0.));
#13319=CARTESIAN_POINT('Ctrl Pts',(8.67274165808153,-1.69485332490039,0.205346305703265));
#13320=CARTESIAN_POINT('Ctrl Pts',(8.66935639350961,-1.68409158103451,0.41069261140653));
#13321=CARTESIAN_POINT('Ctrl Pts',(8.6659711289377,-1.67332983716862,0.616038917109795));
#13322=CARTESIAN_POINT('Ctrl Pts',(4.48443904223854,-1.60211086545473,0.));
#13323=CARTESIAN_POINT('Ctrl Pts',(4.48788860665674,-1.59134912158884,0.205346305703265));
#13324=CARTESIAN_POINT('Ctrl Pts',(4.49133817107494,-1.58058737772296,0.41069261140653));
#13325=CARTESIAN_POINT('Ctrl Pts',(4.49478773549313,-1.56982563385707,0.616038917109795));
#13326=CARTESIAN_POINT('Ctrl Pts',(0.292751161823634,-1.50665779898694,
0.));
#13327=CARTESIAN_POINT('Ctrl Pts',(0.303035555231945,-1.49589605512106,
0.205346305703265));
#13328=CARTESIAN_POINT('Ctrl Pts',(0.313319948640256,-1.48513431125517,
0.41069261140653));
#13329=CARTESIAN_POINT('Ctrl Pts',(0.323604342048567,-1.47437256738929,
0.616038917109795));
#13330=CARTESIAN_POINT('Origin',(0.,-1.5,0.));
#13331=CARTESIAN_POINT('Origin',(6.87409734069396,-2.22044604925031E-16,
0.9));
#13332=CARTESIAN_POINT('Ctrl Pts',(0.292751161823634,1.50665779898694,0.));
#13333=CARTESIAN_POINT('Ctrl Pts',(0.303035555231945,1.49589605512106,0.205346305703265));
#13334=CARTESIAN_POINT('Ctrl Pts',(0.313319948640256,1.48513431125517,0.41069261140653));
#13335=CARTESIAN_POINT('Ctrl Pts',(0.323604342048567,1.47437256738929,0.616038917109795));
#13336=CARTESIAN_POINT('Ctrl Pts',(4.48443904223854,1.60211086545473,0.));
#13337=CARTESIAN_POINT('Ctrl Pts',(4.48788860665674,1.59134912158884,0.205346305703265));
#13338=CARTESIAN_POINT('Ctrl Pts',(4.49133817107493,1.58058737772296,0.41069261140653));
#13339=CARTESIAN_POINT('Ctrl Pts',(4.49478773549313,1.56982563385707,0.616038917109795));
#13340=CARTESIAN_POINT('Ctrl Pts',(8.67612692265345,1.70561506876628,0.));
#13341=CARTESIAN_POINT('Ctrl Pts',(8.67274165808153,1.69485332490039,0.205346305703265));
#13342=CARTESIAN_POINT('Ctrl Pts',(8.66935639350961,1.68409158103451,0.41069261140653));
#13343=CARTESIAN_POINT('Ctrl Pts',(8.66597112893769,1.67332983716862,0.616038917109795));
#13344=CARTESIAN_POINT('Ctrl Pts',(12.8678148030684,2.16300527278356,0.));
#13345=CARTESIAN_POINT('Ctrl Pts',(12.8575947095063,2.15224352891768,0.205346305703265));
#13346=CARTESIAN_POINT('Ctrl Pts',(12.8473746159443,2.14148178505179,0.41069261140653));
#13347=CARTESIAN_POINT('Ctrl Pts',(12.8371545223823,2.13072004118591,0.616038917109795));
#13348=CARTESIAN_POINT('Origin',(13.2,2.2,0.));
#19072=UNCERTAINTY_MEASURE_WITH_UNIT(LENGTH_MEASURE(0.001),#19091,
'DISTANCE_ACCURACY_VALUE',
'Maximum model space distance between geometric entities at asserted c
onnectivities');
#19077=UNCERTAINTY_MEASURE_WITH_UNIT(LENGTH_MEASURE(0.001),#19091,
'DISTANCE_ACCURACY_VALUE',
'Maximum model space distance between geometric entities at asserted c
onnectivities');
#19085=(
GEOMETRIC_REPRESENTATION_CONTEXT(3)
GLOBAL_UNCERTAINTY_ASSIGNED_CONTEXT((#19072))
GLOBAL_UNIT_ASSIGNED_CONTEXT((#19091,#19093,#19094))
REPRESENTATION_CONTEXT('','3D')
);
#19090=(
GEOMETRIC_REPRESENTATION_CONTEXT(3)
GLOBAL_UNCERTAINTY_ASSIGNED_CONTEXT((#19077))
GLOBAL_UNIT_ASSIGNED_CONTEXT((#19091,#19093,#19094))
REPRESENTATION_CONTEXT('','3D')
);
#19091=(
LENGTH_UNIT()
NAMED_UNIT(*)
SI_UNIT(.CENTI.,.METRE.)
);
#19093=(
NAMED_UNIT(*)
PLANE_ANGLE_UNIT()
SI_UNIT($,.RADIAN.)
);
#19094=(
NAMED_UNIT(*)
SI_UNIT($,.STERADIAN.)
SOLID_ANGLE_UNIT()
);
#19102=SHAPE_DEFINITION_REPRESENTATION(#19114,#19142);
#19114=PRODUCT_DEFINITION_SHAPE('',$,#19155);
#19142=SHAPE_REPRESENTATION('',(#7143),#19085);
#19147=PRODUCT_DEFINITION_CONTEXT('part definition',#19185,'design');
#19155=PRODUCT_DEFINITION('2026-11-10-05-09-19-258',
'Lower structural shell',#19167,#19147);
#19167=PRODUCT_DEFINITION_FORMATION('',$,#19194);
#19185=APPLICATION_CONTEXT(
'Core Data for Automotive Mechanical Design Process');
#19186=PRODUCT_CONTEXT('part definition',#19185,'mechanical');
#19194=PRODUCT('2026-11-10-05-09-19-258','Lower structural shell',$,(#19186));
#19203=PRESENTATION_STYLE_ASSIGNMENT((#19211));
#19211=SURFACE_STYLE_USAGE(.BOTH.,#19219);
#19219=SURFACE_SIDE_STYLE('',(#19227));
#19227=SURFACE_STYLE_FILL_AREA(#19235);
#19235=FILL_AREA_STYLE('Structural dark blue',(#19243));
#19243=FILL_AREA_STYLE_COLOUR('Structural dark blue',#19251);
#19251=COLOUR_RGB('Structural dark blue',0.0901960784313725,0.270588235294118,
0.513725490196078);
ENDSEC;
END-ISO-10303-21;
